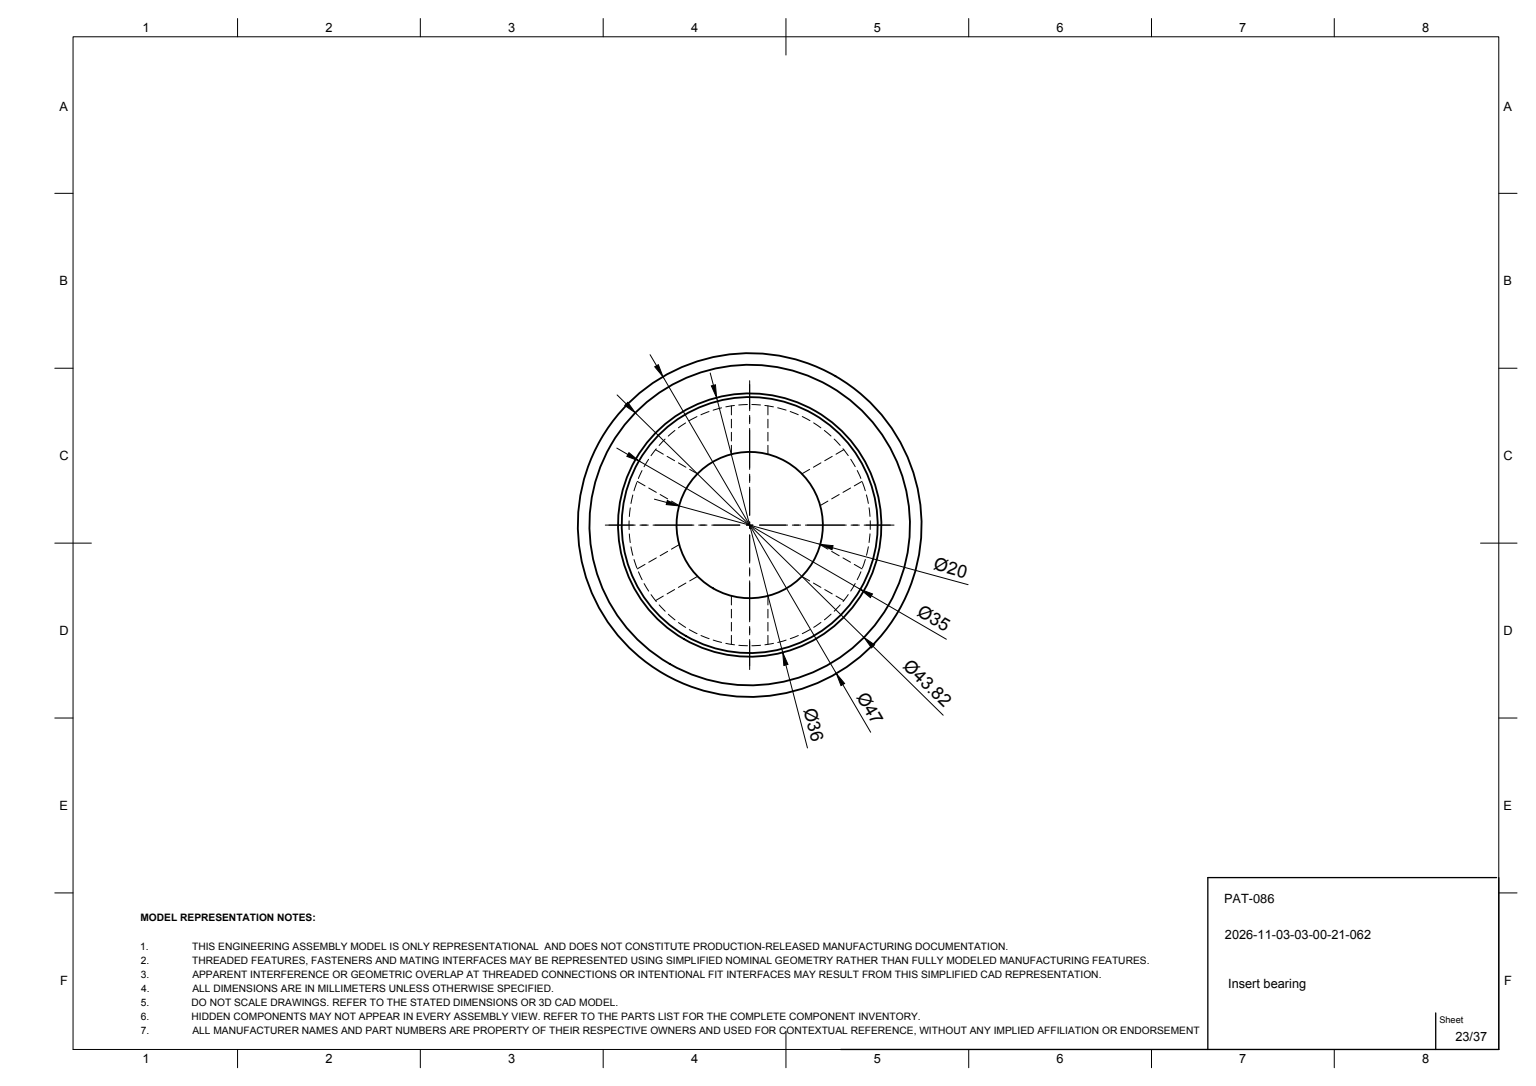
ISO-10303-21;
HEADER;
/* Generated by software containing ST-Developer
 * from STEP Tools, Inc. (www.steptools.com) 
 */

FILE_DESCRIPTION(
/* description */ ('Ratchet and pawl hand winch drum'),
/* implementation_level */ '2;1');

FILE_NAME(
/* name */ 'Insert bearing.step',
/* time_stamp */ '2026-10-27T12:42:58-07:00',
/* author */ (''),
/* organization */ (''),
/* preprocessor_version */ 'ST-DEVELOPER v20.2',
/* originating_system */ 'Autodesk Translation Framework v15.17.0.0',
/* authorisation */ '');

FILE_SCHEMA (('AUTOMOTIVE_DESIGN { 1 0 10303 214 3 1 1 }'));
ENDSEC;

DATA;
#10=MECHANICAL_DESIGN_GEOMETRIC_PRESENTATION_REPRESENTATION('',(#405,#406),#11801);
#273=B_SPLINE_CURVE_WITH_KNOTS('',3,(#9945,#9946,#9947,#9948,#9949,#9950,
#9951,#9952,#9953,#9954),.UNSPECIFIED.,.F.,.F.,(4,2,2,2,4),(1.13193471301885,
1.22626174930539,1.32058878559194,1.41491753480854,1.50924628402513),
 .UNSPECIFIED.);
#274=B_SPLINE_CURVE_WITH_KNOTS('',3,(#9956,#9957,#9958,#9959,#9960,#9961,
#9962,#9963,#9964,#9965,#9966,#9967,#9968,#9969,#9970,#9971,#9972,#9973),
 .UNSPECIFIED.,.F.,.F.,(4,2,2,2,2,2,2,2,4),(0.377311571006283,0.471638607292829,
0.565965643579376,0.66029439279597,0.754623142012565,0.84895189122916,0.943280640445754,
1.0376076767323,1.13193471301885),.UNSPECIFIED.);
#275=B_SPLINE_CURVE_WITH_KNOTS('',3,(#9974,#9975,#9976,#9977,#9978,#9979,
#9980,#9981,#9982,#9983),.UNSPECIFIED.,.F.,.F.,(4,2,2,2,4),(1.50924628402513,
1.60357503324173,1.69790378245832,1.79223081874487,1.88655785503141),
 .UNSPECIFIED.);
#276=B_SPLINE_CURVE_WITH_KNOTS('',3,(#9986,#9987,#9988,#9989,#9990,#9991,
#9992,#9993,#9994,#9995,#9996,#9997,#9998,#9999,#10000,#10001,#10002,#10003,
#10004,#10005,#10006,#10007,#10008,#10009,#10010,#10011,#10012,#10013,#10014,
#10015,#10016,#10017,#10018,#10019),.UNSPECIFIED.,.T.,.F.,(4,2,2,2,2,2,
2,2,2,2,2,2,2,2,2,2,4),(0.,0.0946120580087934,0.189224116017587,0.283822945575014,
0.378421775132442,0.47302060468987,0.567619434247297,0.662231492256091,
0.756843550264884,0.851455608273677,0.94606766628247,1.0406664958399,1.13526532539733,
1.22986415495475,1.32446298451218,1.41907504252097,1.51368710052977),
 .UNSPECIFIED.);
#277=B_SPLINE_CURVE_WITH_KNOTS('',3,(#10022,#10023,#10024,#10025,#10026,
#10027,#10028,#10029,#10030,#10031,#10032,#10033,#10034,#10035,#10036,#10037,
#10038,#10039,#10040,#10041,#10042,#10043,#10044,#10045,#10046,#10047,#10048,
#10049,#10050,#10051,#10052,#10053,#10054,#10055),.UNSPECIFIED.,.T.,.F.,
(4,2,2,2,2,2,2,2,2,2,2,2,2,2,2,2,4),(0.,0.0946120580087934,0.189224116017587,
0.283822945575014,0.378421775132442,0.47302060468987,0.567619434247297,
0.66223149225609,0.756843550264884,0.851455608273677,0.94606766628247,1.0406664958399,
1.13526532539733,1.22986415495475,1.32446298451218,1.41907504252097,1.51368710052977),
 .UNSPECIFIED.);
#278=B_SPLINE_CURVE_WITH_KNOTS('',3,(#10059,#10060,#10061,#10062,#10063,
#10064,#10065,#10066,#10067,#10068),.UNSPECIFIED.,.F.,.F.,(4,2,2,2,4),(1.13193471301885,
1.22626174930539,1.32058878559194,1.41491753480854,1.50924628402513),
 .UNSPECIFIED.);
#279=B_SPLINE_CURVE_WITH_KNOTS('',3,(#10070,#10071,#10072,#10073,#10074,
#10075,#10076,#10077,#10078,#10079,#10080,#10081,#10082,#10083,#10084,#10085,
#10086,#10087),.UNSPECIFIED.,.F.,.F.,(4,2,2,2,2,2,2,2,4),(0.377311571006283,
0.47163860729283,0.565965643579376,0.660294392795971,0.754623142012565,
0.84895189122916,0.943280640445755,1.0376076767323,1.13193471301885),
 .UNSPECIFIED.);
#280=B_SPLINE_CURVE_WITH_KNOTS('',3,(#10088,#10089,#10090,#10091,#10092,
#10093,#10094,#10095,#10096,#10097),.UNSPECIFIED.,.F.,.F.,(4,2,2,2,4),(1.50924628402513,
1.60357503324173,1.69790378245832,1.79223081874487,1.88655785503141),
 .UNSPECIFIED.);
#281=B_SPLINE_CURVE_WITH_KNOTS('',3,(#10106,#10107,#10108,#10109,#10110,
#10111,#10112,#10113,#10114,#10115,#10116,#10117,#10118,#10119,#10120,#10121,
#10122,#10123),.UNSPECIFIED.,.F.,.F.,(4,2,2,2,2,2,2,2,4),(0.377311571006282,
0.471638607292829,0.565965643579376,0.660294392795971,0.754623142012565,
0.84895189122916,0.943280640445754,1.0376076767323,1.13193471301885),
 .UNSPECIFIED.);
#282=B_SPLINE_CURVE_WITH_KNOTS('',3,(#10125,#10126,#10127,#10128,#10129,
#10130,#10131,#10132,#10133,#10134),.UNSPECIFIED.,.F.,.F.,(4,2,2,2,4),(1.13193471301885,
1.22626174930539,1.32058878559194,1.41491753480854,1.50924628402513),
 .UNSPECIFIED.);
#283=B_SPLINE_CURVE_WITH_KNOTS('',3,(#10135,#10136,#10137,#10138,#10139,
#10140,#10141,#10142,#10143,#10144),.UNSPECIFIED.,.F.,.F.,(4,2,2,2,4),(1.50924628402513,
1.60357503324172,1.69790378245832,1.79223081874487,1.88655785503141),
 .UNSPECIFIED.);
#284=B_SPLINE_CURVE_WITH_KNOTS('',3,(#10147,#10148,#10149,#10150,#10151,
#10152,#10153,#10154,#10155,#10156,#10157,#10158,#10159,#10160,#10161,#10162,
#10163,#10164),.UNSPECIFIED.,.F.,.F.,(4,2,2,2,2,2,2,2,4),(0.377311571006283,
0.47163860729283,0.565965643579376,0.660294392795971,0.754623142012565,
0.84895189122916,0.943280640445754,1.0376076767323,1.13193471301885),
 .UNSPECIFIED.);
#285=B_SPLINE_CURVE_WITH_KNOTS('',3,(#10166,#10167,#10168,#10169,#10170,
#10171,#10172,#10173,#10174,#10175),.UNSPECIFIED.,.F.,.F.,(4,2,2,2,4),(1.13193471301885,
1.22626174930539,1.32058878559194,1.41491753480854,1.50924628402513),
 .UNSPECIFIED.);
#286=B_SPLINE_CURVE_WITH_KNOTS('',3,(#10176,#10177,#10178,#10179,#10180,
#10181,#10182,#10183,#10184,#10185),.UNSPECIFIED.,.F.,.F.,(4,2,2,2,4),(1.50924628402513,
1.60357503324173,1.69790378245832,1.79223081874487,1.88655785503141),
 .UNSPECIFIED.);
#287=B_SPLINE_CURVE_WITH_KNOTS('',3,(#10188,#10189,#10190,#10191,#10192,
#10193,#10194,#10195,#10196,#10197,#10198,#10199,#10200,#10201,#10202,#10203,
#10204,#10205),.UNSPECIFIED.,.F.,.F.,(4,2,2,2,2,2,2,2,4),(0.377311571006282,
0.471638607292829,0.565965643579376,0.66029439279597,0.754623142012565,
0.84895189122916,0.943280640445754,1.0376076767323,1.13193471301885),
 .UNSPECIFIED.);
#288=B_SPLINE_CURVE_WITH_KNOTS('',3,(#10207,#10208,#10209,#10210,#10211,
#10212,#10213,#10214,#10215,#10216),.UNSPECIFIED.,.F.,.F.,(4,2,2,2,4),(1.13193471301885,
1.22626174930539,1.32058878559194,1.41491753480854,1.50924628402513),
 .UNSPECIFIED.);
#289=B_SPLINE_CURVE_WITH_KNOTS('',3,(#10217,#10218,#10219,#10220,#10221,
#10222,#10223,#10224,#10225,#10226),.UNSPECIFIED.,.F.,.F.,(4,2,2,2,4),(1.50924628402513,
1.60357503324172,1.69790378245832,1.79223081874487,1.88655785503141),
 .UNSPECIFIED.);
#290=B_SPLINE_CURVE_WITH_KNOTS('',3,(#10229,#10230,#10231,#10232,#10233,
#10234,#10235,#10236,#10237,#10238,#10239,#10240,#10241,#10242,#10243,#10244,
#10245,#10246),.UNSPECIFIED.,.F.,.F.,(4,2,2,2,2,2,2,2,4),(0.377311571006283,
0.471638607292829,0.565965643579376,0.660294392795971,0.754623142012565,
0.84895189122916,0.943280640445755,1.0376076767323,1.13193471301885),
 .UNSPECIFIED.);
#291=B_SPLINE_CURVE_WITH_KNOTS('',3,(#10248,#10249,#10250,#10251,#10252,
#10253,#10254,#10255,#10256,#10257),.UNSPECIFIED.,.F.,.F.,(4,2,2,2,4),(1.13193471301885,
1.22626174930539,1.32058878559194,1.41491753480854,1.50924628402513),
 .UNSPECIFIED.);
#292=B_SPLINE_CURVE_WITH_KNOTS('',3,(#10258,#10259,#10260,#10261,#10262,
#10263,#10264,#10265,#10266,#10267),.UNSPECIFIED.,.F.,.F.,(4,2,2,2,4),(1.50924628402513,
1.60357503324172,1.69790378245832,1.79223081874487,1.88655785503141),
 .UNSPECIFIED.);
#293=B_SPLINE_CURVE_WITH_KNOTS('',3,(#10271,#10272,#10273,#10274,#10275,
#10276,#10277,#10278,#10279,#10280,#10281,#10282,#10283,#10284,#10285,#10286,
#10287,#10288,#10289,#10290,#10291,#10292,#10293,#10294,#10295,#10296,#10297,
#10298,#10299,#10300,#10301,#10302,#10303,#10304),.UNSPECIFIED.,.T.,.F.,
(4,2,2,2,2,2,2,2,2,2,2,2,2,2,2,2,4),(0.,0.0946120580087934,0.189224116017587,
0.283822945575014,0.378421775132442,0.47302060468987,0.567619434247297,
0.66223149225609,0.756843550264884,0.851455608273677,0.94606766628247,1.0406664958399,
1.13526532539733,1.22986415495475,1.32446298451218,1.41907504252097,1.51368710052977),
 .UNSPECIFIED.);
#294=B_SPLINE_CURVE_WITH_KNOTS('',3,(#10307,#10308,#10309,#10310,#10311,
#10312,#10313,#10314,#10315,#10316,#10317,#10318,#10319,#10320,#10321,#10322,
#10323,#10324,#10325,#10326,#10327,#10328,#10329,#10330,#10331,#10332,#10333,
#10334,#10335,#10336,#10337,#10338,#10339,#10340),.UNSPECIFIED.,.T.,.F.,
(4,2,2,2,2,2,2,2,2,2,2,2,2,2,2,2,4),(0.,0.0946120580087934,0.189224116017587,
0.283822945575014,0.378421775132442,0.47302060468987,0.567619434247297,
0.66223149225609,0.756843550264884,0.851455608273677,0.94606766628247,1.0406664958399,
1.13526532539733,1.22986415495475,1.32446298451218,1.41907504252097,1.51368710052977),
 .UNSPECIFIED.);
#295=B_SPLINE_CURVE_WITH_KNOTS('',3,(#10345,#10346,#10347,#10348,#10349,
#10350,#10351,#10352,#10353,#10354,#10355,#10356,#10357,#10358,#10359,#10360,
#10361,#10362,#10363,#10364,#10365,#10366,#10367,#10368,#10369,#10370,#10371,
#10372,#10373,#10374,#10375,#10376,#10377,#10378),.UNSPECIFIED.,.T.,.F.,
(4,2,2,2,2,2,2,2,2,2,2,2,2,2,2,2,4),(0.,0.0946120580087934,0.189224116017587,
0.283822945575014,0.378421775132442,0.47302060468987,0.567619434247297,
0.66223149225609,0.756843550264884,0.851455608273677,0.94606766628247,1.0406664958399,
1.13526532539733,1.22986415495475,1.32446298451218,1.41907504252097,1.51368710052977),
 .UNSPECIFIED.);
#296=B_SPLINE_CURVE_WITH_KNOTS('',3,(#10381,#10382,#10383,#10384,#10385,
#10386,#10387,#10388,#10389,#10390,#10391,#10392,#10393,#10394,#10395,#10396,
#10397,#10398,#10399,#10400,#10401,#10402,#10403,#10404,#10405,#10406,#10407,
#10408,#10409,#10410,#10411,#10412,#10413,#10414),.UNSPECIFIED.,.T.,.F.,
(4,2,2,2,2,2,2,2,2,2,2,2,2,2,2,2,4),(0.,0.0946120580087934,0.189224116017587,
0.283822945575014,0.378421775132442,0.47302060468987,0.567619434247297,
0.66223149225609,0.756843550264884,0.851455608273677,0.94606766628247,1.0406664958399,
1.13526532539733,1.22986415495475,1.32446298451218,1.41907504252097,1.51368710052977),
 .UNSPECIFIED.);
#320=SPHERICAL_SURFACE('',#6968,2.35);
#337=SHAPE_REPRESENTATION_RELATIONSHIP('SRR','None',#11964,#371);
#371=ADVANCED_BREP_SHAPE_REPRESENTATION('',(#440,#441),#11781);
#405=STYLED_ITEM('',(#12213),#440);
#406=STYLED_ITEM('',(#12213),#441);
#440=MANIFOLD_SOLID_BREP('Body1',#6282);
#441=MANIFOLD_SOLID_BREP('Body2',#6283);
#541=FACE_BOUND('',#1434,.T.);
#542=FACE_BOUND('',#1436,.T.);
#543=FACE_BOUND('',#1437,.T.);
#544=FACE_BOUND('',#1439,.T.);
#545=FACE_BOUND('',#1443,.T.);
#546=FACE_BOUND('',#1444,.T.);
#547=FACE_BOUND('',#1445,.T.);
#548=FACE_BOUND('',#1446,.T.);
#549=FACE_BOUND('',#1447,.T.);
#550=FACE_BOUND('',#1448,.T.);
#551=FACE_BOUND('',#1454,.T.);
#552=FACE_BOUND('',#1456,.T.);
#553=FACE_BOUND('',#1459,.T.);
#554=FACE_BOUND('',#1461,.T.);
#555=FACE_BOUND('',#1462,.T.);
#556=FACE_BOUND('',#1463,.T.);
#557=FACE_BOUND('',#1464,.T.);
#558=FACE_BOUND('',#1465,.T.);
#559=FACE_BOUND('',#1466,.T.);
#697=PLANE('',#6966);
#698=PLANE('',#6971);
#699=PLANE('',#6981);
#700=PLANE('',#6983);
#701=PLANE('',#6987);
#991=FACE_OUTER_BOUND('',#1432,.T.);
#992=FACE_OUTER_BOUND('',#1433,.T.);
#993=FACE_OUTER_BOUND('',#1435,.T.);
#994=FACE_OUTER_BOUND('',#1438,.T.);
#995=FACE_OUTER_BOUND('',#1440,.T.);
#996=FACE_OUTER_BOUND('',#1441,.T.);
#997=FACE_OUTER_BOUND('',#1442,.T.);
#998=FACE_OUTER_BOUND('',#1449,.T.);
#999=FACE_OUTER_BOUND('',#1450,.T.);
#1000=FACE_OUTER_BOUND('',#1451,.T.);
#1001=FACE_OUTER_BOUND('',#1452,.T.);
#1002=FACE_OUTER_BOUND('',#1453,.T.);
#1003=FACE_OUTER_BOUND('',#1455,.T.);
#1004=FACE_OUTER_BOUND('',#1457,.T.);
#1005=FACE_OUTER_BOUND('',#1458,.T.);
#1006=FACE_OUTER_BOUND('',#1460,.T.);
#1432=EDGE_LOOP('',(#4879,#4880,#4881,#4882));
#1433=EDGE_LOOP('',(#4883));
#1434=EDGE_LOOP('',(#4884));
#1435=EDGE_LOOP('',(#4885,#4886));
#1436=EDGE_LOOP('',(#4887));
#1437=EDGE_LOOP('',(#4888));
#1438=EDGE_LOOP('',(#4889));
#1439=EDGE_LOOP('',(#4890));
#1440=EDGE_LOOP('',(#4891,#4892,#4893,#4894,#4895,#4896));
#1441=EDGE_LOOP('',(#4897,#4898,#4899,#4900,#4901,#4902));
#1442=EDGE_LOOP('',(#4903,#4904,#4905,#4906));
#1443=EDGE_LOOP('',(#4907,#4908,#4909));
#1444=EDGE_LOOP('',(#4910,#4911,#4912));
#1445=EDGE_LOOP('',(#4913,#4914,#4915));
#1446=EDGE_LOOP('',(#4916,#4917,#4918));
#1447=EDGE_LOOP('',(#4919,#4920,#4921));
#1448=EDGE_LOOP('',(#4922,#4923,#4924));
#1449=EDGE_LOOP('',(#4925,#4926,#4927,#4928,#4929,#4930));
#1450=EDGE_LOOP('',(#4931,#4932,#4933,#4934,#4935,#4936));
#1451=EDGE_LOOP('',(#4937,#4938,#4939,#4940,#4941,#4942));
#1452=EDGE_LOOP('',(#4943,#4944,#4945,#4946,#4947,#4948));
#1453=EDGE_LOOP('',(#4949));
#1454=EDGE_LOOP('',(#4950));
#1455=EDGE_LOOP('',(#4951));
#1456=EDGE_LOOP('',(#4952));
#1457=EDGE_LOOP('',(#4953,#4954,#4955,#4956));
#1458=EDGE_LOOP('',(#4957));
#1459=EDGE_LOOP('',(#4958));
#1460=EDGE_LOOP('',(#4959,#4960,#4961,#4962));
#1461=EDGE_LOOP('',(#4963));
#1462=EDGE_LOOP('',(#4964));
#1463=EDGE_LOOP('',(#4965));
#1464=EDGE_LOOP('',(#4966));
#1465=EDGE_LOOP('',(#4967));
#1466=EDGE_LOOP('',(#4968));
#1900=LINE('',#9930,#2411);
#1901=LINE('',#9985,#2412);
#1902=LINE('',#10057,#2413);
#1903=LINE('',#10102,#2414);
#1904=LINE('',#10270,#2415);
#1905=LINE('',#10341,#2416);
#1906=LINE('',#10344,#2417);
#1907=LINE('',#10415,#2418);
#1908=LINE('',#10425,#2419);
#1909=LINE('',#10430,#2420);
#2411=VECTOR('',#8133,1.8);
#2412=VECTOR('',#8150,0.25);
#2413=VECTOR('',#8153,0.25);
#2414=VECTOR('',#8158,1.65);
#2415=VECTOR('',#8163,0.25);
#2416=VECTOR('',#8166,0.25);
#2417=VECTOR('',#8169,0.25);
#2418=VECTOR('',#8172,0.25);
#2419=VECTOR('',#8185,1.75);
#2420=VECTOR('',#8192,1.);
#2832=CIRCLE('',#6964,1.8);
#2833=CIRCLE('',#6965,1.8);
#2834=CIRCLE('',#6967,2.19089023002066);
#2835=CIRCLE('',#6969,2.35);
#2836=CIRCLE('',#6970,2.19089023002066);
#2837=CIRCLE('',#6975,1.65);
#2838=CIRCLE('',#6976,1.65);
#2839=CIRCLE('',#6982,1.);
#2840=CIRCLE('',#6984,1.75);
#2841=CIRCLE('',#6986,1.75);
#2842=CIRCLE('',#6988,1.);
#3154=VERTEX_POINT('',#9927);
#3155=VERTEX_POINT('',#9929);
#3156=VERTEX_POINT('',#9933);
#3157=VERTEX_POINT('',#9936);
#3158=VERTEX_POINT('',#9937);
#3159=VERTEX_POINT('',#9939);
#3160=VERTEX_POINT('',#9943);
#3161=VERTEX_POINT('',#9944);
#3162=VERTEX_POINT('',#9955);
#3163=VERTEX_POINT('',#9984);
#3164=VERTEX_POINT('',#10021);
#3165=VERTEX_POINT('',#10056);
#3166=VERTEX_POINT('',#10058);
#3167=VERTEX_POINT('',#10069);
#3168=VERTEX_POINT('',#10099);
#3169=VERTEX_POINT('',#10101);
#3170=VERTEX_POINT('',#10104);
#3171=VERTEX_POINT('',#10105);
#3172=VERTEX_POINT('',#10124);
#3173=VERTEX_POINT('',#10145);
#3174=VERTEX_POINT('',#10146);
#3175=VERTEX_POINT('',#10165);
#3176=VERTEX_POINT('',#10186);
#3177=VERTEX_POINT('',#10187);
#3178=VERTEX_POINT('',#10206);
#3179=VERTEX_POINT('',#10227);
#3180=VERTEX_POINT('',#10228);
#3181=VERTEX_POINT('',#10247);
#3182=VERTEX_POINT('',#10269);
#3183=VERTEX_POINT('',#10306);
#3184=VERTEX_POINT('',#10343);
#3185=VERTEX_POINT('',#10380);
#3186=VERTEX_POINT('',#10417);
#3187=VERTEX_POINT('',#10420);
#3188=VERTEX_POINT('',#10423);
#3189=VERTEX_POINT('',#10427);
#3783=EDGE_CURVE('',#3154,#3154,#2832,.T.);
#3784=EDGE_CURVE('',#3154,#3155,#1900,.T.);
#3785=EDGE_CURVE('',#3155,#3155,#2833,.T.);
#3786=EDGE_CURVE('',#3156,#3156,#2834,.T.);
#3787=EDGE_CURVE('',#3157,#3158,#2835,.T.);
#3788=EDGE_CURVE('',#3159,#3159,#2836,.T.);
#3789=EDGE_CURVE('',#3160,#3161,#273,.T.);
#3790=EDGE_CURVE('',#3162,#3160,#274,.T.);
#3791=EDGE_CURVE('',#3161,#3162,#275,.T.);
#3792=EDGE_CURVE('',#3161,#3163,#1901,.T.);
#3793=EDGE_CURVE('',#3163,#3163,#276,.T.);
#3794=EDGE_CURVE('',#3164,#3164,#277,.T.);
#3795=EDGE_CURVE('',#3164,#3165,#1902,.T.);
#3796=EDGE_CURVE('',#3166,#3165,#278,.T.);
#3797=EDGE_CURVE('',#3167,#3166,#279,.T.);
#3798=EDGE_CURVE('',#3165,#3167,#280,.T.);
#3799=EDGE_CURVE('',#3168,#3168,#2837,.T.);
#3800=EDGE_CURVE('',#3168,#3169,#1903,.T.);
#3801=EDGE_CURVE('',#3169,#3169,#2838,.T.);
#3802=EDGE_CURVE('',#3170,#3171,#281,.T.);
#3803=EDGE_CURVE('',#3171,#3172,#282,.T.);
#3804=EDGE_CURVE('',#3172,#3170,#283,.T.);
#3805=EDGE_CURVE('',#3173,#3174,#284,.T.);
#3806=EDGE_CURVE('',#3174,#3175,#285,.T.);
#3807=EDGE_CURVE('',#3175,#3173,#286,.T.);
#3808=EDGE_CURVE('',#3176,#3177,#287,.T.);
#3809=EDGE_CURVE('',#3177,#3178,#288,.T.);
#3810=EDGE_CURVE('',#3178,#3176,#289,.T.);
#3811=EDGE_CURVE('',#3179,#3180,#290,.T.);
#3812=EDGE_CURVE('',#3180,#3181,#291,.T.);
#3813=EDGE_CURVE('',#3181,#3179,#292,.T.);
#3814=EDGE_CURVE('',#3172,#3182,#1904,.T.);
#3815=EDGE_CURVE('',#3182,#3182,#293,.T.);
#3816=EDGE_CURVE('',#3183,#3183,#294,.T.);
#3817=EDGE_CURVE('',#3183,#3175,#1905,.T.);
#3818=EDGE_CURVE('',#3178,#3184,#1906,.T.);
#3819=EDGE_CURVE('',#3184,#3184,#295,.T.);
#3820=EDGE_CURVE('',#3185,#3185,#296,.T.);
#3821=EDGE_CURVE('',#3185,#3181,#1907,.T.);
#3822=EDGE_CURVE('',#3186,#3186,#2839,.T.);
#3823=EDGE_CURVE('',#3187,#3187,#2840,.T.);
#3824=EDGE_CURVE('',#3188,#3188,#2841,.T.);
#3825=EDGE_CURVE('',#3188,#3187,#1908,.T.);
#3826=EDGE_CURVE('',#3189,#3189,#2842,.T.);
#3827=EDGE_CURVE('',#3189,#3186,#1909,.T.);
#4879=ORIENTED_EDGE('',*,*,#3783,.T.);
#4880=ORIENTED_EDGE('',*,*,#3784,.T.);
#4881=ORIENTED_EDGE('',*,*,#3785,.F.);
#4882=ORIENTED_EDGE('',*,*,#3784,.F.);
#4883=ORIENTED_EDGE('',*,*,#3786,.F.);
#4884=ORIENTED_EDGE('',*,*,#3785,.T.);
#4885=ORIENTED_EDGE('',*,*,#3787,.T.);
#4886=ORIENTED_EDGE('',*,*,#3787,.F.);
#4887=ORIENTED_EDGE('',*,*,#3786,.T.);
#4888=ORIENTED_EDGE('',*,*,#3788,.F.);
#4889=ORIENTED_EDGE('',*,*,#3788,.T.);
#4890=ORIENTED_EDGE('',*,*,#3783,.F.);
#4891=ORIENTED_EDGE('',*,*,#3789,.F.);
#4892=ORIENTED_EDGE('',*,*,#3790,.F.);
#4893=ORIENTED_EDGE('',*,*,#3791,.F.);
#4894=ORIENTED_EDGE('',*,*,#3792,.T.);
#4895=ORIENTED_EDGE('',*,*,#3793,.F.);
#4896=ORIENTED_EDGE('',*,*,#3792,.F.);
#4897=ORIENTED_EDGE('',*,*,#3794,.F.);
#4898=ORIENTED_EDGE('',*,*,#3795,.T.);
#4899=ORIENTED_EDGE('',*,*,#3796,.F.);
#4900=ORIENTED_EDGE('',*,*,#3797,.F.);
#4901=ORIENTED_EDGE('',*,*,#3798,.F.);
#4902=ORIENTED_EDGE('',*,*,#3795,.F.);
#4903=ORIENTED_EDGE('',*,*,#3799,.F.);
#4904=ORIENTED_EDGE('',*,*,#3800,.T.);
#4905=ORIENTED_EDGE('',*,*,#3801,.T.);
#4906=ORIENTED_EDGE('',*,*,#3800,.F.);
#4907=ORIENTED_EDGE('',*,*,#3790,.T.);
#4908=ORIENTED_EDGE('',*,*,#3789,.T.);
#4909=ORIENTED_EDGE('',*,*,#3791,.T.);
#4910=ORIENTED_EDGE('',*,*,#3797,.T.);
#4911=ORIENTED_EDGE('',*,*,#3796,.T.);
#4912=ORIENTED_EDGE('',*,*,#3798,.T.);
#4913=ORIENTED_EDGE('',*,*,#3802,.T.);
#4914=ORIENTED_EDGE('',*,*,#3803,.T.);
#4915=ORIENTED_EDGE('',*,*,#3804,.T.);
#4916=ORIENTED_EDGE('',*,*,#3805,.T.);
#4917=ORIENTED_EDGE('',*,*,#3806,.T.);
#4918=ORIENTED_EDGE('',*,*,#3807,.T.);
#4919=ORIENTED_EDGE('',*,*,#3808,.T.);
#4920=ORIENTED_EDGE('',*,*,#3809,.T.);
#4921=ORIENTED_EDGE('',*,*,#3810,.T.);
#4922=ORIENTED_EDGE('',*,*,#3811,.T.);
#4923=ORIENTED_EDGE('',*,*,#3812,.T.);
#4924=ORIENTED_EDGE('',*,*,#3813,.T.);
#4925=ORIENTED_EDGE('',*,*,#3803,.F.);
#4926=ORIENTED_EDGE('',*,*,#3802,.F.);
#4927=ORIENTED_EDGE('',*,*,#3804,.F.);
#4928=ORIENTED_EDGE('',*,*,#3814,.T.);
#4929=ORIENTED_EDGE('',*,*,#3815,.F.);
#4930=ORIENTED_EDGE('',*,*,#3814,.F.);
#4931=ORIENTED_EDGE('',*,*,#3816,.F.);
#4932=ORIENTED_EDGE('',*,*,#3817,.T.);
#4933=ORIENTED_EDGE('',*,*,#3806,.F.);
#4934=ORIENTED_EDGE('',*,*,#3805,.F.);
#4935=ORIENTED_EDGE('',*,*,#3807,.F.);
#4936=ORIENTED_EDGE('',*,*,#3817,.F.);
#4937=ORIENTED_EDGE('',*,*,#3809,.F.);
#4938=ORIENTED_EDGE('',*,*,#3808,.F.);
#4939=ORIENTED_EDGE('',*,*,#3810,.F.);
#4940=ORIENTED_EDGE('',*,*,#3818,.T.);
#4941=ORIENTED_EDGE('',*,*,#3819,.F.);
#4942=ORIENTED_EDGE('',*,*,#3818,.F.);
#4943=ORIENTED_EDGE('',*,*,#3820,.F.);
#4944=ORIENTED_EDGE('',*,*,#3821,.T.);
#4945=ORIENTED_EDGE('',*,*,#3812,.F.);
#4946=ORIENTED_EDGE('',*,*,#3811,.F.);
#4947=ORIENTED_EDGE('',*,*,#3813,.F.);
#4948=ORIENTED_EDGE('',*,*,#3821,.F.);
#4949=ORIENTED_EDGE('',*,*,#3801,.F.);
#4950=ORIENTED_EDGE('',*,*,#3822,.T.);
#4951=ORIENTED_EDGE('',*,*,#3823,.F.);
#4952=ORIENTED_EDGE('',*,*,#3799,.T.);
#4953=ORIENTED_EDGE('',*,*,#3824,.F.);
#4954=ORIENTED_EDGE('',*,*,#3825,.T.);
#4955=ORIENTED_EDGE('',*,*,#3823,.T.);
#4956=ORIENTED_EDGE('',*,*,#3825,.F.);
#4957=ORIENTED_EDGE('',*,*,#3824,.T.);
#4958=ORIENTED_EDGE('',*,*,#3826,.F.);
#4959=ORIENTED_EDGE('',*,*,#3826,.T.);
#4960=ORIENTED_EDGE('',*,*,#3827,.T.);
#4961=ORIENTED_EDGE('',*,*,#3822,.F.);
#4962=ORIENTED_EDGE('',*,*,#3827,.F.);
#4963=ORIENTED_EDGE('',*,*,#3794,.T.);
#4964=ORIENTED_EDGE('',*,*,#3793,.T.);
#4965=ORIENTED_EDGE('',*,*,#3816,.T.);
#4966=ORIENTED_EDGE('',*,*,#3815,.T.);
#4967=ORIENTED_EDGE('',*,*,#3820,.T.);
#4968=ORIENTED_EDGE('',*,*,#3819,.T.);
#5861=CYLINDRICAL_SURFACE('',#6963,1.8);
#5862=CYLINDRICAL_SURFACE('',#6972,0.25);
#5863=CYLINDRICAL_SURFACE('',#6973,0.25);
#5864=CYLINDRICAL_SURFACE('',#6974,1.65);
#5865=CYLINDRICAL_SURFACE('',#6977,0.25);
#5866=CYLINDRICAL_SURFACE('',#6978,0.25);
#5867=CYLINDRICAL_SURFACE('',#6979,0.25);
#5868=CYLINDRICAL_SURFACE('',#6980,0.25);
#5869=CYLINDRICAL_SURFACE('',#6985,1.75);
#5870=CYLINDRICAL_SURFACE('',#6989,1.);
#6061=ADVANCED_FACE('',(#991),#5861,.F.);
#6062=ADVANCED_FACE('',(#992,#541),#697,.T.);
#6063=ADVANCED_FACE('',(#993,#542,#543),#320,.T.);
#6064=ADVANCED_FACE('',(#994,#544),#698,.T.);
#6065=ADVANCED_FACE('',(#995),#5862,.F.);
#6066=ADVANCED_FACE('',(#996),#5863,.F.);
#6067=ADVANCED_FACE('',(#997,#545,#546,#547,#548,#549,#550),#5864,.T.);
#6068=ADVANCED_FACE('',(#998),#5865,.F.);
#6069=ADVANCED_FACE('',(#999),#5866,.F.);
#6070=ADVANCED_FACE('',(#1000),#5867,.F.);
#6071=ADVANCED_FACE('',(#1001),#5868,.F.);
#6072=ADVANCED_FACE('',(#1002,#551),#699,.T.);
#6073=ADVANCED_FACE('',(#1003,#552),#700,.T.);
#6074=ADVANCED_FACE('',(#1004),#5869,.T.);
#6075=ADVANCED_FACE('',(#1005,#553),#701,.T.);
#6076=ADVANCED_FACE('',(#1006,#554,#555,#556,#557,#558,#559),#5870,.F.);
#6282=CLOSED_SHELL('',(#6061,#6062,#6063,#6064));
#6283=CLOSED_SHELL('',(#6065,#6066,#6067,#6068,#6069,#6070,#6071,#6072,
#6073,#6074,#6075,#6076));
#6962=AXIS2_PLACEMENT_3D('',#9925,#8127,#8128);
#6963=AXIS2_PLACEMENT_3D('',#9926,#8129,#8130);
#6964=AXIS2_PLACEMENT_3D('',#9928,#8131,#8132);
#6965=AXIS2_PLACEMENT_3D('',#9931,#8134,#8135);
#6966=AXIS2_PLACEMENT_3D('',#9932,#8136,#8137);
#6967=AXIS2_PLACEMENT_3D('',#9934,#8138,#8139);
#6968=AXIS2_PLACEMENT_3D('',#9935,#8140,#8141);
#6969=AXIS2_PLACEMENT_3D('',#9938,#8142,#8143);
#6970=AXIS2_PLACEMENT_3D('',#9940,#8144,#8145);
#6971=AXIS2_PLACEMENT_3D('',#9941,#8146,#8147);
#6972=AXIS2_PLACEMENT_3D('',#9942,#8148,#8149);
#6973=AXIS2_PLACEMENT_3D('',#10020,#8151,#8152);
#6974=AXIS2_PLACEMENT_3D('',#10098,#8154,#8155);
#6975=AXIS2_PLACEMENT_3D('',#10100,#8156,#8157);
#6976=AXIS2_PLACEMENT_3D('',#10103,#8159,#8160);
#6977=AXIS2_PLACEMENT_3D('',#10268,#8161,#8162);
#6978=AXIS2_PLACEMENT_3D('',#10305,#8164,#8165);
#6979=AXIS2_PLACEMENT_3D('',#10342,#8167,#8168);
#6980=AXIS2_PLACEMENT_3D('',#10379,#8170,#8171);
#6981=AXIS2_PLACEMENT_3D('',#10416,#8173,#8174);
#6982=AXIS2_PLACEMENT_3D('',#10418,#8175,#8176);
#6983=AXIS2_PLACEMENT_3D('',#10419,#8177,#8178);
#6984=AXIS2_PLACEMENT_3D('',#10421,#8179,#8180);
#6985=AXIS2_PLACEMENT_3D('',#10422,#8181,#8182);
#6986=AXIS2_PLACEMENT_3D('',#10424,#8183,#8184);
#6987=AXIS2_PLACEMENT_3D('',#10426,#8186,#8187);
#6988=AXIS2_PLACEMENT_3D('',#10428,#8188,#8189);
#6989=AXIS2_PLACEMENT_3D('',#10429,#8190,#8191);
#8127=DIRECTION('axis',(0.,0.,1.));
#8128=DIRECTION('refdir',(1.,0.,0.));
#8129=DIRECTION('center_axis',(0.,-1.,0.));
#8130=DIRECTION('ref_axis',(1.,0.,0.));
#8131=DIRECTION('center_axis',(0.,-1.,0.));
#8132=DIRECTION('ref_axis',(1.,0.,0.));
#8133=DIRECTION('',(0.,1.,0.));
#8134=DIRECTION('center_axis',(0.,-1.,0.));
#8135=DIRECTION('ref_axis',(1.,0.,0.));
#8136=DIRECTION('center_axis',(0.,1.,0.));
#8137=DIRECTION('ref_axis',(0.,0.,1.));
#8138=DIRECTION('center_axis',(0.,-1.,0.));
#8139=DIRECTION('ref_axis',(1.,0.,0.));
#8140=DIRECTION('center_axis',(6.12323399573677E-17,0.,1.));
#8141=DIRECTION('ref_axis',(1.,0.,0.));
#8142=DIRECTION('center_axis',(1.22464679914735E-16,-1.,0.));
#8143=DIRECTION('ref_axis',(-1.,-1.22464679914735E-16,0.));
#8144=DIRECTION('center_axis',(0.,-1.,0.));
#8145=DIRECTION('ref_axis',(1.,0.,0.));
#8146=DIRECTION('center_axis',(0.,-1.,0.));
#8147=DIRECTION('ref_axis',(0.,0.,-1.));
#8148=DIRECTION('center_axis',(-0.866025403784438,0.,-0.5));
#8149=DIRECTION('ref_axis',(-0.5,0.,0.866025403784438));
#8150=DIRECTION('',(-0.866025403784438,0.,-0.5));
#8151=DIRECTION('center_axis',(-0.866025403784438,0.,-0.5));
#8152=DIRECTION('ref_axis',(-0.5,0.,0.866025403784438));
#8153=DIRECTION('',(-0.866025403784438,0.,-0.5));
#8154=DIRECTION('center_axis',(0.,-1.,0.));
#8155=DIRECTION('ref_axis',(1.,0.,0.));
#8156=DIRECTION('center_axis',(0.,-1.,0.));
#8157=DIRECTION('ref_axis',(1.,0.,0.));
#8158=DIRECTION('',(0.,1.,0.));
#8159=DIRECTION('center_axis',(0.,-1.,0.));
#8160=DIRECTION('ref_axis',(1.,0.,0.));
#8161=DIRECTION('center_axis',(0.866025403784439,0.,-0.5));
#8162=DIRECTION('ref_axis',(-0.5,0.,-0.866025403784439));
#8163=DIRECTION('',(0.866025403784439,0.,-0.5));
#8164=DIRECTION('center_axis',(0.866025403784439,0.,-0.5));
#8165=DIRECTION('ref_axis',(-0.5,0.,-0.866025403784439));
#8166=DIRECTION('',(0.866025403784439,0.,-0.5));
#8167=DIRECTION('center_axis',(0.,0.,1.));
#8168=DIRECTION('ref_axis',(1.,0.,0.));
#8169=DIRECTION('',(0.,0.,1.));
#8170=DIRECTION('center_axis',(0.,0.,1.));
#8171=DIRECTION('ref_axis',(1.,0.,0.));
#8172=DIRECTION('',(0.,0.,1.));
#8173=DIRECTION('center_axis',(0.,1.,0.));
#8174=DIRECTION('ref_axis',(0.,0.,1.));
#8175=DIRECTION('center_axis',(0.,-1.,0.));
#8176=DIRECTION('ref_axis',(1.,0.,0.));
#8177=DIRECTION('center_axis',(0.,1.,0.));
#8178=DIRECTION('ref_axis',(0.,0.,1.));
#8179=DIRECTION('center_axis',(0.,-1.,0.));
#8180=DIRECTION('ref_axis',(1.,0.,0.));
#8181=DIRECTION('center_axis',(0.,-1.,0.));
#8182=DIRECTION('ref_axis',(1.,0.,0.));
#8183=DIRECTION('center_axis',(0.,-1.,0.));
#8184=DIRECTION('ref_axis',(1.,0.,0.));
#8185=DIRECTION('',(0.,1.,0.));
#8186=DIRECTION('center_axis',(0.,-1.,0.));
#8187=DIRECTION('ref_axis',(0.,0.,-1.));
#8188=DIRECTION('center_axis',(0.,-1.,0.));
#8189=DIRECTION('ref_axis',(1.,0.,0.));
#8190=DIRECTION('center_axis',(0.,-1.,0.));
#8191=DIRECTION('ref_axis',(1.,0.,0.));
#8192=DIRECTION('',(0.,1.,0.));
#9925=CARTESIAN_POINT('',(0.,0.,0.));
#9926=CARTESIAN_POINT('Origin',(0.,0.,0.));
#9927=CARTESIAN_POINT('',(-1.8,-0.85,-2.20436423846524E-16));
#9928=CARTESIAN_POINT('Origin',(0.,-0.85,0.));
#9929=CARTESIAN_POINT('',(-1.8,0.85,-2.20436423846524E-16));
#9930=CARTESIAN_POINT('',(-1.8,0.,-2.20436423846524E-16));
#9931=CARTESIAN_POINT('Origin',(0.,0.85,0.));
#9932=CARTESIAN_POINT('Origin',(2.19089023002066,0.85,0.));
#9933=CARTESIAN_POINT('',(2.19089023002066,0.85,0.));
#9934=CARTESIAN_POINT('Origin',(0.,0.85,0.));
#9935=CARTESIAN_POINT('Origin',(3.99680288865056E-15,0.,0.));
#9936=CARTESIAN_POINT('',(3.85290688975075E-15,-1.76221774462768E-32,2.35));
#9937=CARTESIAN_POINT('',(3.85290688975075E-15,-1.76221774462768E-32,-2.35));
#9938=CARTESIAN_POINT('Origin',(3.99680288865056E-15,0.,0.));
#9939=CARTESIAN_POINT('',(2.19089023002066,-0.85,0.));
#9940=CARTESIAN_POINT('Origin',(0.,-0.85,0.));
#9941=CARTESIAN_POINT('Origin',(1.8,-0.85,0.));
#9942=CARTESIAN_POINT('Origin',(0.,1.55,0.));
#9943=CARTESIAN_POINT('',(1.42894191624432,1.8,0.825000000000001));
#9944=CARTESIAN_POINT('',(1.53744468918255,1.55,0.598968970568896));
#9945=CARTESIAN_POINT('Ctrl Pts',(1.42894191624432,1.8,0.825000000000001));
#9946=CARTESIAN_POINT('Ctrl Pts',(1.44466308895875,1.8,0.797770130104052));
#9947=CARTESIAN_POINT('Ctrl Pts',(1.46055812562105,1.79370633789704,0.768258557763732));
#9948=CARTESIAN_POINT('Ctrl Pts',(1.48824888379079,1.76817777258318,0.713138492740816));
#9949=CARTESIAN_POINT('Ctrl Pts',(1.50008999307766,1.74894552961493,0.687551581002689));
#9950=CARTESIAN_POINT('Ctrl Pts',(1.51812136280714,1.70460745840382,0.646764802471699));
#9951=CARTESIAN_POINT('Ctrl Pts',(1.52552758004446,1.67652816181843,0.628833667319578));
#9952=CARTESIAN_POINT('Ctrl Pts',(1.53516661651472,1.61494799959182,0.604921184808251));
#9953=CARTESIAN_POINT('Ctrl Pts',(1.53744468918255,1.58144291640553,0.598968970568896));
#9954=CARTESIAN_POINT('Ctrl Pts',(1.53744468918255,1.55,0.598968970568896));
#9955=CARTESIAN_POINT('',(1.42894191624432,1.3,0.825000000000001));
#9956=CARTESIAN_POINT('Ctrl Pts',(1.42894191624432,1.3,0.825000000000001));
#9957=CARTESIAN_POINT('Ctrl Pts',(1.4132207435299,1.3,0.852229869895949));
#9958=CARTESIAN_POINT('Ctrl Pts',(1.39561049050871,1.30629366210296,0.880751161609749));
#9959=CARTESIAN_POINT('Ctrl Pts',(1.36172049302549,1.33182222741682,0.932292094146256));
#9960=CARTESIAN_POINT('Ctrl Pts',(1.34548213209931,1.35105447038507,0.955340251466734));
#9961=CARTESIAN_POINT('Ctrl Pts',(1.31917543061769,1.39539254159618,0.99134926498299));
#9962=CARTESIAN_POINT('Ctrl Pts',(1.30734972067592,1.42347183818157,1.00672880483252));
#9963=CARTESIAN_POINT('Ctrl Pts',(1.29146042158868,1.48505200040818,1.02703269653942));
#9964=CARTESIAN_POINT('Ctrl Pts',(1.28744468918255,1.51855708359447,1.03198167246111));
#9965=CARTESIAN_POINT('Ctrl Pts',(1.28744468918255,1.58144291640553,1.03198167246111));
#9966=CARTESIAN_POINT('Ctrl Pts',(1.29146042158868,1.61494799959182,1.02703269653942));
#9967=CARTESIAN_POINT('Ctrl Pts',(1.30734972067592,1.67652816181843,1.00672880483252));
#9968=CARTESIAN_POINT('Ctrl Pts',(1.31917543061769,1.70460745840382,0.991349264982991));
#9969=CARTESIAN_POINT('Ctrl Pts',(1.34548213209931,1.74894552961493,0.955340251466735));
#9970=CARTESIAN_POINT('Ctrl Pts',(1.36172049302549,1.76817777258318,0.932292094146256));
#9971=CARTESIAN_POINT('Ctrl Pts',(1.39561049050871,1.79370633789704,0.880751161609749));
#9972=CARTESIAN_POINT('Ctrl Pts',(1.4132207435299,1.8,0.85222986989595));
#9973=CARTESIAN_POINT('Ctrl Pts',(1.42894191624432,1.8,0.825000000000001));
#9974=CARTESIAN_POINT('Ctrl Pts',(1.53744468918255,1.55,0.598968970568896));
#9975=CARTESIAN_POINT('Ctrl Pts',(1.53744468918255,1.51855708359447,0.598968970568896));
#9976=CARTESIAN_POINT('Ctrl Pts',(1.53516661651472,1.48505200040818,0.60492118480825));
#9977=CARTESIAN_POINT('Ctrl Pts',(1.52552758004446,1.42347183818157,0.628833667319578));
#9978=CARTESIAN_POINT('Ctrl Pts',(1.51812136280714,1.39539254159618,0.646764802471699));
#9979=CARTESIAN_POINT('Ctrl Pts',(1.50008999307766,1.35105447038507,0.687551581002689));
#9980=CARTESIAN_POINT('Ctrl Pts',(1.48824888379079,1.33182222741682,0.713138492740816));
#9981=CARTESIAN_POINT('Ctrl Pts',(1.46055812562105,1.30629366210296,0.768258557763732));
#9982=CARTESIAN_POINT('Ctrl Pts',(1.44466308895875,1.3,0.797770130104052));
#9983=CARTESIAN_POINT('Ctrl Pts',(1.42894191624432,1.3,0.825000000000001));
#9984=CARTESIAN_POINT('',(0.963525491562421,1.55,0.267616567329818));
#9985=CARTESIAN_POINT('',(0.125,1.55,-0.21650635094611));
#9986=CARTESIAN_POINT('Ctrl Pts',(0.963525491562421,1.55,0.267616567329818));
#9987=CARTESIAN_POINT('Ctrl Pts',(0.963525491562421,1.5815373526696,0.267616567329818));
#9988=CARTESIAN_POINT('Ctrl Pts',(0.961833761492987,1.61508042700263,0.273949373987484));
#9989=CARTESIAN_POINT('Ctrl Pts',(0.954308486908894,1.67663267125761,0.299111603474268));
#9990=CARTESIAN_POINT('Ctrl Pts',(0.948394987258249,1.70465411363682,0.31788699900678));
#9991=CARTESIAN_POINT('Ctrl Pts',(0.933155485613026,1.74889618382539,0.360174810895352));
#9992=CARTESIAN_POINT('Ctrl Pts',(0.92278792026947,1.76811531482682,0.386546956384144));
#9993=CARTESIAN_POINT('Ctrl Pts',(0.897143218189782,1.79367084275751,0.442820664919227));
#9994=CARTESIAN_POINT('Ctrl Pts',(0.881791875377343,1.8,0.472691670144998));
#9995=CARTESIAN_POINT('Ctrl Pts',(0.850258932191534,1.8,0.527308329855003));
#9996=CARTESIAN_POINT('Ctrl Pts',(0.832065554235658,1.79367084275751,0.555538485325664));
#9997=CARTESIAN_POINT('Ctrl Pts',(0.796153444118959,1.76811531482682,0.605884303066698));
#9998=CARTESIAN_POINT('Ctrl Pts',(0.778498278845144,1.74889618382539,0.62804895077401));
#9999=CARTESIAN_POINT('Ctrl Pts',(0.749495710301794,1.70465411363682,0.662390652284073));
#10000=CARTESIAN_POINT('Ctrl Pts',(0.73619249062986,1.67663267125761,0.676899590973058));
#10001=CARTESIAN_POINT('Ctrl Pts',(0.718163997970498,1.61508042700263,0.695997784676728));
#10002=CARTESIAN_POINT('Ctrl Pts',(0.713525491562421,1.5815373526696,0.700629269222037));
#10003=CARTESIAN_POINT('Ctrl Pts',(0.713525491562421,1.5184626473304,0.700629269222037));
#10004=CARTESIAN_POINT('Ctrl Pts',(0.718163997970498,1.48491957299737,0.695997784676728));
#10005=CARTESIAN_POINT('Ctrl Pts',(0.73619249062986,1.42336732874239,0.676899590973058));
#10006=CARTESIAN_POINT('Ctrl Pts',(0.749495710301794,1.39534588636318,0.662390652284073));
#10007=CARTESIAN_POINT('Ctrl Pts',(0.778498278845144,1.35110381617461,0.62804895077401));
#10008=CARTESIAN_POINT('Ctrl Pts',(0.796153444118959,1.33188468517318,0.605884303066698));
#10009=CARTESIAN_POINT('Ctrl Pts',(0.832065554235658,1.30632915724249,0.555538485325664));
#10010=CARTESIAN_POINT('Ctrl Pts',(0.850258932191534,1.3,0.527308329855003));
#10011=CARTESIAN_POINT('Ctrl Pts',(0.881791875377343,1.3,0.472691670144998));
#10012=CARTESIAN_POINT('Ctrl Pts',(0.897143218189782,1.30632915724249,0.442820664919227));
#10013=CARTESIAN_POINT('Ctrl Pts',(0.92278792026947,1.33188468517318,0.386546956384144));
#10014=CARTESIAN_POINT('Ctrl Pts',(0.933155485613026,1.35110381617461,0.360174810895352));
#10015=CARTESIAN_POINT('Ctrl Pts',(0.948394987258249,1.39534588636318,0.31788699900678));
#10016=CARTESIAN_POINT('Ctrl Pts',(0.954308486908894,1.42336732874239,0.299111603474268));
#10017=CARTESIAN_POINT('Ctrl Pts',(0.961833761492987,1.48491957299738,0.273949373987484));
#10018=CARTESIAN_POINT('Ctrl Pts',(0.963525491562421,1.5184626473304,0.267616567329818));
#10019=CARTESIAN_POINT('Ctrl Pts',(0.963525491562421,1.55,0.267616567329818));
#10020=CARTESIAN_POINT('Origin',(0.,1.55,0.));
#10021=CARTESIAN_POINT('',(-0.713525491562421,1.55,-0.700629269222037));
#10022=CARTESIAN_POINT('Ctrl Pts',(-0.713525491562421,1.55,-0.700629269222037));
#10023=CARTESIAN_POINT('Ctrl Pts',(-0.713525491562421,1.5184626473304,-0.700629269222037));
#10024=CARTESIAN_POINT('Ctrl Pts',(-0.718163997970498,1.48491957299737,
-0.695997784676728));
#10025=CARTESIAN_POINT('Ctrl Pts',(-0.73619249062986,1.42336732874239,-0.676899590973058));
#10026=CARTESIAN_POINT('Ctrl Pts',(-0.749495710301794,1.39534588636318,
-0.662390652284073));
#10027=CARTESIAN_POINT('Ctrl Pts',(-0.778498278845144,1.35110381617461,
-0.62804895077401));
#10028=CARTESIAN_POINT('Ctrl Pts',(-0.796153444118959,1.33188468517318,
-0.605884303066698));
#10029=CARTESIAN_POINT('Ctrl Pts',(-0.832065554235658,1.30632915724249,
-0.555538485325664));
#10030=CARTESIAN_POINT('Ctrl Pts',(-0.850258932191534,1.3,-0.527308329855003));
#10031=CARTESIAN_POINT('Ctrl Pts',(-0.881791875377343,1.3,-0.472691670144998));
#10032=CARTESIAN_POINT('Ctrl Pts',(-0.897143218189782,1.30632915724249,
-0.442820664919227));
#10033=CARTESIAN_POINT('Ctrl Pts',(-0.92278792026947,1.33188468517318,-0.386546956384144));
#10034=CARTESIAN_POINT('Ctrl Pts',(-0.933155485613026,1.35110381617461,
-0.360174810895352));
#10035=CARTESIAN_POINT('Ctrl Pts',(-0.948394987258249,1.39534588636318,
-0.31788699900678));
#10036=CARTESIAN_POINT('Ctrl Pts',(-0.954308486908894,1.42336732874239,
-0.299111603474268));
#10037=CARTESIAN_POINT('Ctrl Pts',(-0.961833761492986,1.48491957299737,
-0.273949373987484));
#10038=CARTESIAN_POINT('Ctrl Pts',(-0.963525491562421,1.5184626473304,-0.267616567329818));
#10039=CARTESIAN_POINT('Ctrl Pts',(-0.963525491562421,1.5815373526696,-0.267616567329818));
#10040=CARTESIAN_POINT('Ctrl Pts',(-0.961833761492986,1.61508042700263,
-0.273949373987484));
#10041=CARTESIAN_POINT('Ctrl Pts',(-0.954308486908894,1.67663267125761,
-0.299111603474268));
#10042=CARTESIAN_POINT('Ctrl Pts',(-0.948394987258249,1.70465411363682,
-0.31788699900678));
#10043=CARTESIAN_POINT('Ctrl Pts',(-0.933155485613026,1.74889618382539,
-0.360174810895352));
#10044=CARTESIAN_POINT('Ctrl Pts',(-0.92278792026947,1.76811531482682,-0.386546956384144));
#10045=CARTESIAN_POINT('Ctrl Pts',(-0.897143218189782,1.79367084275751,
-0.442820664919227));
#10046=CARTESIAN_POINT('Ctrl Pts',(-0.881791875377343,1.8,-0.472691670144998));
#10047=CARTESIAN_POINT('Ctrl Pts',(-0.850258932191534,1.8,-0.527308329855003));
#10048=CARTESIAN_POINT('Ctrl Pts',(-0.832065554235658,1.79367084275751,
-0.555538485325664));
#10049=CARTESIAN_POINT('Ctrl Pts',(-0.796153444118959,1.76811531482682,
-0.605884303066698));
#10050=CARTESIAN_POINT('Ctrl Pts',(-0.778498278845144,1.74889618382539,
-0.62804895077401));
#10051=CARTESIAN_POINT('Ctrl Pts',(-0.749495710301794,1.70465411363682,
-0.662390652284073));
#10052=CARTESIAN_POINT('Ctrl Pts',(-0.73619249062986,1.67663267125761,-0.676899590973058));
#10053=CARTESIAN_POINT('Ctrl Pts',(-0.718163997970498,1.61508042700263,
-0.695997784676728));
#10054=CARTESIAN_POINT('Ctrl Pts',(-0.713525491562421,1.5815373526696,-0.700629269222037));
#10055=CARTESIAN_POINT('Ctrl Pts',(-0.713525491562421,1.55,-0.700629269222037));
#10056=CARTESIAN_POINT('',(-1.28744468918255,1.55,-1.03198167246111));
#10057=CARTESIAN_POINT('',(0.125,1.55,-0.21650635094611));
#10058=CARTESIAN_POINT('',(-1.42894191624432,1.3,-0.825000000000001));
#10059=CARTESIAN_POINT('Ctrl Pts',(-1.42894191624432,1.3,-0.825000000000001));
#10060=CARTESIAN_POINT('Ctrl Pts',(-1.4132207435299,1.3,-0.852229869895949));
#10061=CARTESIAN_POINT('Ctrl Pts',(-1.39561049050871,1.30629366210296,-0.880751161609749));
#10062=CARTESIAN_POINT('Ctrl Pts',(-1.36172049302549,1.33182222741682,-0.932292094146256));
#10063=CARTESIAN_POINT('Ctrl Pts',(-1.34548213209931,1.35105447038507,-0.955340251466735));
#10064=CARTESIAN_POINT('Ctrl Pts',(-1.31917543061769,1.39539254159618,-0.991349264982991));
#10065=CARTESIAN_POINT('Ctrl Pts',(-1.30734972067592,1.42347183818157,-1.00672880483252));
#10066=CARTESIAN_POINT('Ctrl Pts',(-1.29146042158868,1.48505200040818,-1.02703269653942));
#10067=CARTESIAN_POINT('Ctrl Pts',(-1.28744468918255,1.51855708359447,-1.03198167246111));
#10068=CARTESIAN_POINT('Ctrl Pts',(-1.28744468918255,1.55,-1.03198167246111));
#10069=CARTESIAN_POINT('',(-1.42894191624432,1.8,-0.825000000000001));
#10070=CARTESIAN_POINT('Ctrl Pts',(-1.42894191624432,1.8,-0.825000000000001));
#10071=CARTESIAN_POINT('Ctrl Pts',(-1.44466308895875,1.8,-0.797770130104052));
#10072=CARTESIAN_POINT('Ctrl Pts',(-1.46055812562105,1.79370633789704,-0.768258557763732));
#10073=CARTESIAN_POINT('Ctrl Pts',(-1.48824888379079,1.76817777258318,-0.713138492740816));
#10074=CARTESIAN_POINT('Ctrl Pts',(-1.50008999307766,1.74894552961493,-0.687551581002689));
#10075=CARTESIAN_POINT('Ctrl Pts',(-1.51812136280714,1.70460745840382,-0.646764802471699));
#10076=CARTESIAN_POINT('Ctrl Pts',(-1.52552758004446,1.67652816181843,-0.628833667319578));
#10077=CARTESIAN_POINT('Ctrl Pts',(-1.53516661651472,1.61494799959182,-0.60492118480825));
#10078=CARTESIAN_POINT('Ctrl Pts',(-1.53744468918255,1.58144291640553,-0.598968970568896));
#10079=CARTESIAN_POINT('Ctrl Pts',(-1.53744468918255,1.51855708359447,-0.598968970568896));
#10080=CARTESIAN_POINT('Ctrl Pts',(-1.53516661651472,1.48505200040818,-0.60492118480825));
#10081=CARTESIAN_POINT('Ctrl Pts',(-1.52552758004446,1.42347183818157,-0.628833667319578));
#10082=CARTESIAN_POINT('Ctrl Pts',(-1.51812136280714,1.39539254159618,-0.646764802471699));
#10083=CARTESIAN_POINT('Ctrl Pts',(-1.50008999307766,1.35105447038507,-0.687551581002689));
#10084=CARTESIAN_POINT('Ctrl Pts',(-1.48824888379079,1.33182222741682,-0.713138492740816));
#10085=CARTESIAN_POINT('Ctrl Pts',(-1.46055812562105,1.30629366210296,-0.768258557763732));
#10086=CARTESIAN_POINT('Ctrl Pts',(-1.44466308895875,1.3,-0.797770130104052));
#10087=CARTESIAN_POINT('Ctrl Pts',(-1.42894191624432,1.3,-0.825000000000001));
#10088=CARTESIAN_POINT('Ctrl Pts',(-1.28744468918255,1.55,-1.03198167246111));
#10089=CARTESIAN_POINT('Ctrl Pts',(-1.28744468918255,1.58144291640553,-1.03198167246111));
#10090=CARTESIAN_POINT('Ctrl Pts',(-1.29146042158868,1.61494799959182,-1.02703269653942));
#10091=CARTESIAN_POINT('Ctrl Pts',(-1.30734972067592,1.67652816181843,-1.00672880483252));
#10092=CARTESIAN_POINT('Ctrl Pts',(-1.31917543061769,1.70460745840382,-0.991349264982991));
#10093=CARTESIAN_POINT('Ctrl Pts',(-1.34548213209931,1.74894552961493,-0.955340251466734));
#10094=CARTESIAN_POINT('Ctrl Pts',(-1.36172049302549,1.76817777258318,-0.932292094146256));
#10095=CARTESIAN_POINT('Ctrl Pts',(-1.39561049050871,1.79370633789704,-0.880751161609749));
#10096=CARTESIAN_POINT('Ctrl Pts',(-1.4132207435299,1.8,-0.852229869895949));
#10097=CARTESIAN_POINT('Ctrl Pts',(-1.42894191624432,1.8,-0.825000000000001));
#10098=CARTESIAN_POINT('Origin',(0.,1.55,0.));
#10099=CARTESIAN_POINT('',(-1.65,0.85,-2.02066721859313E-16));
#10100=CARTESIAN_POINT('Origin',(0.,0.85,0.));
#10101=CARTESIAN_POINT('',(-1.65,2.25,-2.02066721859313E-16));
#10102=CARTESIAN_POINT('',(-1.65,1.55,-2.02066721859313E-16));
#10103=CARTESIAN_POINT('Origin',(0.,2.25,0.));
#10104=CARTESIAN_POINT('',(-1.42894191624432,1.3,0.825));
#10105=CARTESIAN_POINT('',(-1.42894191624432,1.8,0.825));
#10106=CARTESIAN_POINT('Ctrl Pts',(-1.42894191624432,1.3,0.825));
#10107=CARTESIAN_POINT('Ctrl Pts',(-1.44466308895875,1.3,0.797770130104051));
#10108=CARTESIAN_POINT('Ctrl Pts',(-1.46055812562105,1.30629366210296,0.768258557763731));
#10109=CARTESIAN_POINT('Ctrl Pts',(-1.48824888379079,1.33182222741682,0.713138492740815));
#10110=CARTESIAN_POINT('Ctrl Pts',(-1.50008999307766,1.35105447038507,0.687551581002688));
#10111=CARTESIAN_POINT('Ctrl Pts',(-1.51812136280714,1.39539254159618,0.646764802471698));
#10112=CARTESIAN_POINT('Ctrl Pts',(-1.52552758004446,1.42347183818157,0.628833667319577));
#10113=CARTESIAN_POINT('Ctrl Pts',(-1.53516661651472,1.48505200040818,0.604921184808249));
#10114=CARTESIAN_POINT('Ctrl Pts',(-1.53744468918255,1.51855708359447,0.598968970568895));
#10115=CARTESIAN_POINT('Ctrl Pts',(-1.53744468918255,1.58144291640553,0.598968970568895));
#10116=CARTESIAN_POINT('Ctrl Pts',(-1.53516661651472,1.61494799959182,0.604921184808249));
#10117=CARTESIAN_POINT('Ctrl Pts',(-1.52552758004446,1.67652816181843,0.628833667319577));
#10118=CARTESIAN_POINT('Ctrl Pts',(-1.51812136280714,1.70460745840382,0.646764802471698));
#10119=CARTESIAN_POINT('Ctrl Pts',(-1.50008999307766,1.74894552961493,0.687551581002688));
#10120=CARTESIAN_POINT('Ctrl Pts',(-1.48824888379079,1.76817777258318,0.713138492740815));
#10121=CARTESIAN_POINT('Ctrl Pts',(-1.46055812562105,1.79370633789704,0.768258557763731));
#10122=CARTESIAN_POINT('Ctrl Pts',(-1.44466308895875,1.8,0.797770130104051));
#10123=CARTESIAN_POINT('Ctrl Pts',(-1.42894191624432,1.8,0.825));
#10124=CARTESIAN_POINT('',(-1.28744468918255,1.55,1.03198167246111));
#10125=CARTESIAN_POINT('Ctrl Pts',(-1.42894191624432,1.8,0.825));
#10126=CARTESIAN_POINT('Ctrl Pts',(-1.4132207435299,1.8,0.852229869895948));
#10127=CARTESIAN_POINT('Ctrl Pts',(-1.39561049050871,1.79370633789704,0.880751161609747));
#10128=CARTESIAN_POINT('Ctrl Pts',(-1.36172049302549,1.76817777258318,0.932292094146255));
#10129=CARTESIAN_POINT('Ctrl Pts',(-1.34548213209931,1.74894552961493,0.955340251466733));
#10130=CARTESIAN_POINT('Ctrl Pts',(-1.31917543061769,1.70460745840382,0.991349264982989));
#10131=CARTESIAN_POINT('Ctrl Pts',(-1.30734972067592,1.67652816181843,1.00672880483252));
#10132=CARTESIAN_POINT('Ctrl Pts',(-1.29146042158868,1.61494799959182,1.02703269653942));
#10133=CARTESIAN_POINT('Ctrl Pts',(-1.28744468918255,1.58144291640553,1.03198167246111));
#10134=CARTESIAN_POINT('Ctrl Pts',(-1.28744468918255,1.55,1.03198167246111));
#10135=CARTESIAN_POINT('Ctrl Pts',(-1.28744468918255,1.55,1.03198167246111));
#10136=CARTESIAN_POINT('Ctrl Pts',(-1.28744468918255,1.51855708359447,1.03198167246111));
#10137=CARTESIAN_POINT('Ctrl Pts',(-1.29146042158868,1.48505200040818,1.02703269653942));
#10138=CARTESIAN_POINT('Ctrl Pts',(-1.30734972067592,1.42347183818157,1.00672880483252));
#10139=CARTESIAN_POINT('Ctrl Pts',(-1.31917543061769,1.39539254159618,0.99134926498299));
#10140=CARTESIAN_POINT('Ctrl Pts',(-1.34548213209931,1.35105447038508,0.955340251466733));
#10141=CARTESIAN_POINT('Ctrl Pts',(-1.36172049302549,1.33182222741682,0.932292094146255));
#10142=CARTESIAN_POINT('Ctrl Pts',(-1.39561049050871,1.30629366210296,0.880751161609748));
#10143=CARTESIAN_POINT('Ctrl Pts',(-1.4132207435299,1.3,0.852229869895949));
#10144=CARTESIAN_POINT('Ctrl Pts',(-1.42894191624432,1.3,0.825));
#10145=CARTESIAN_POINT('',(1.42894191624432,1.8,-0.825));
#10146=CARTESIAN_POINT('',(1.42894191624432,1.3,-0.825));
#10147=CARTESIAN_POINT('Ctrl Pts',(1.42894191624432,1.8,-0.825));
#10148=CARTESIAN_POINT('Ctrl Pts',(1.4132207435299,1.8,-0.852229869895949));
#10149=CARTESIAN_POINT('Ctrl Pts',(1.39561049050871,1.79370633789704,-0.880751161609748));
#10150=CARTESIAN_POINT('Ctrl Pts',(1.36172049302549,1.76817777258318,-0.932292094146255));
#10151=CARTESIAN_POINT('Ctrl Pts',(1.34548213209931,1.74894552961493,-0.955340251466734));
#10152=CARTESIAN_POINT('Ctrl Pts',(1.31917543061769,1.70460745840382,-0.99134926498299));
#10153=CARTESIAN_POINT('Ctrl Pts',(1.30734972067592,1.67652816181843,-1.00672880483252));
#10154=CARTESIAN_POINT('Ctrl Pts',(1.29146042158868,1.61494799959182,-1.02703269653942));
#10155=CARTESIAN_POINT('Ctrl Pts',(1.28744468918255,1.58144291640553,-1.03198167246111));
#10156=CARTESIAN_POINT('Ctrl Pts',(1.28744468918255,1.51855708359447,-1.03198167246111));
#10157=CARTESIAN_POINT('Ctrl Pts',(1.29146042158868,1.48505200040818,-1.02703269653942));
#10158=CARTESIAN_POINT('Ctrl Pts',(1.30734972067592,1.42347183818157,-1.00672880483252));
#10159=CARTESIAN_POINT('Ctrl Pts',(1.31917543061769,1.39539254159618,-0.99134926498299));
#10160=CARTESIAN_POINT('Ctrl Pts',(1.34548213209931,1.35105447038507,-0.955340251466734));
#10161=CARTESIAN_POINT('Ctrl Pts',(1.36172049302549,1.33182222741682,-0.932292094146255));
#10162=CARTESIAN_POINT('Ctrl Pts',(1.39561049050871,1.30629366210296,-0.880751161609748));
#10163=CARTESIAN_POINT('Ctrl Pts',(1.4132207435299,1.3,-0.852229869895948));
#10164=CARTESIAN_POINT('Ctrl Pts',(1.42894191624432,1.3,-0.825));
#10165=CARTESIAN_POINT('',(1.53744468918255,1.55,-0.598968970568895));
#10166=CARTESIAN_POINT('Ctrl Pts',(1.42894191624432,1.3,-0.825));
#10167=CARTESIAN_POINT('Ctrl Pts',(1.44466308895875,1.3,-0.797770130104051));
#10168=CARTESIAN_POINT('Ctrl Pts',(1.46055812562105,1.30629366210296,-0.768258557763731));
#10169=CARTESIAN_POINT('Ctrl Pts',(1.48824888379079,1.33182222741682,-0.713138492740815));
#10170=CARTESIAN_POINT('Ctrl Pts',(1.50008999307766,1.35105447038507,-0.687551581002688));
#10171=CARTESIAN_POINT('Ctrl Pts',(1.51812136280714,1.39539254159618,-0.646764802471698));
#10172=CARTESIAN_POINT('Ctrl Pts',(1.52552758004446,1.42347183818157,-0.628833667319577));
#10173=CARTESIAN_POINT('Ctrl Pts',(1.53516661651472,1.48505200040818,-0.604921184808249));
#10174=CARTESIAN_POINT('Ctrl Pts',(1.53744468918255,1.51855708359447,-0.598968970568895));
#10175=CARTESIAN_POINT('Ctrl Pts',(1.53744468918255,1.55,-0.598968970568895));
#10176=CARTESIAN_POINT('Ctrl Pts',(1.53744468918255,1.55,-0.598968970568895));
#10177=CARTESIAN_POINT('Ctrl Pts',(1.53744468918255,1.58144291640553,-0.598968970568895));
#10178=CARTESIAN_POINT('Ctrl Pts',(1.53516661651472,1.61494799959182,-0.604921184808249));
#10179=CARTESIAN_POINT('Ctrl Pts',(1.52552758004446,1.67652816181843,-0.628833667319577));
#10180=CARTESIAN_POINT('Ctrl Pts',(1.51812136280714,1.70460745840382,-0.646764802471698));
#10181=CARTESIAN_POINT('Ctrl Pts',(1.50008999307766,1.74894552961493,-0.687551581002688));
#10182=CARTESIAN_POINT('Ctrl Pts',(1.48824888379079,1.76817777258318,-0.713138492740815));
#10183=CARTESIAN_POINT('Ctrl Pts',(1.46055812562105,1.79370633789704,-0.768258557763731));
#10184=CARTESIAN_POINT('Ctrl Pts',(1.44466308895875,1.8,-0.797770130104051));
#10185=CARTESIAN_POINT('Ctrl Pts',(1.42894191624432,1.8,-0.825));
#10186=CARTESIAN_POINT('',(0.,1.3,-1.65));
#10187=CARTESIAN_POINT('',(0.,1.8,-1.65));
#10188=CARTESIAN_POINT('Ctrl Pts',(1.38777878078145E-17,1.3,-1.65));
#10189=CARTESIAN_POINT('Ctrl Pts',(0.0314423454288489,1.3,-1.65));
#10190=CARTESIAN_POINT('Ctrl Pts',(0.0649476351123396,1.30629366210296,
-1.64900971937348));
#10191=CARTESIAN_POINT('Ctrl Pts',(0.126528390765307,1.33182222741682,-1.64543058688707));
#10192=CARTESIAN_POINT('Ctrl Pts',(0.154607860978348,1.35105447038507,-1.64289183246942));
#10193=CARTESIAN_POINT('Ctrl Pts',(0.198945932189457,1.39539254159618,-1.63811406745469));
#10194=CARTESIAN_POINT('Ctrl Pts',(0.218177859368546,1.42347183818157,-1.63556247215209));
#10195=CARTESIAN_POINT('Ctrl Pts',(0.243706194926033,1.48505200040818,-1.63195388134767));
#10196=CARTESIAN_POINT('Ctrl Pts',(0.25,1.51855708359447,-1.63095064303001));
#10197=CARTESIAN_POINT('Ctrl Pts',(0.25,1.58144291640553,-1.63095064303001));
#10198=CARTESIAN_POINT('Ctrl Pts',(0.243706194926033,1.61494799959182,-1.63195388134767));
#10199=CARTESIAN_POINT('Ctrl Pts',(0.218177859368546,1.67652816181843,-1.63556247215209));
#10200=CARTESIAN_POINT('Ctrl Pts',(0.198945932189457,1.70460745840382,-1.63811406745469));
#10201=CARTESIAN_POINT('Ctrl Pts',(0.154607860978349,1.74894552961493,-1.64289183246942));
#10202=CARTESIAN_POINT('Ctrl Pts',(0.126528390765307,1.76817777258318,-1.64543058688707));
#10203=CARTESIAN_POINT('Ctrl Pts',(0.0649476351123398,1.79370633789704,
-1.64900971937348));
#10204=CARTESIAN_POINT('Ctrl Pts',(0.031442345428849,1.8,-1.65));
#10205=CARTESIAN_POINT('Ctrl Pts',(7.63278329429795E-17,1.8,-1.65));
#10206=CARTESIAN_POINT('',(-0.25,1.55,-1.63095064303001));
#10207=CARTESIAN_POINT('Ctrl Pts',(9.0205620750794E-17,1.8,-1.65));
#10208=CARTESIAN_POINT('Ctrl Pts',(-0.0314423454288488,1.8,-1.65));
#10209=CARTESIAN_POINT('Ctrl Pts',(-0.0649476351123396,1.79370633789704,
-1.64900971937348));
#10210=CARTESIAN_POINT('Ctrl Pts',(-0.126528390765307,1.76817777258318,
-1.64543058688707));
#10211=CARTESIAN_POINT('Ctrl Pts',(-0.154607860978348,1.74894552961493,
-1.64289183246942));
#10212=CARTESIAN_POINT('Ctrl Pts',(-0.198945932189456,1.70460745840382,
-1.63811406745469));
#10213=CARTESIAN_POINT('Ctrl Pts',(-0.218177859368546,1.67652816181843,
-1.63556247215209));
#10214=CARTESIAN_POINT('Ctrl Pts',(-0.243706194926033,1.61494799959182,
-1.63195388134767));
#10215=CARTESIAN_POINT('Ctrl Pts',(-0.25,1.58144291640553,-1.63095064303001));
#10216=CARTESIAN_POINT('Ctrl Pts',(-0.25,1.55,-1.63095064303001));
#10217=CARTESIAN_POINT('Ctrl Pts',(-0.25,1.55,-1.63095064303001));
#10218=CARTESIAN_POINT('Ctrl Pts',(-0.25,1.51855708359447,-1.63095064303001));
#10219=CARTESIAN_POINT('Ctrl Pts',(-0.243706194926033,1.48505200040818,
-1.63195388134767));
#10220=CARTESIAN_POINT('Ctrl Pts',(-0.218177859368546,1.42347183818157,
-1.63556247215209));
#10221=CARTESIAN_POINT('Ctrl Pts',(-0.198945932189457,1.39539254159618,
-1.63811406745469));
#10222=CARTESIAN_POINT('Ctrl Pts',(-0.154607860978349,1.35105447038507,
-1.64289183246942));
#10223=CARTESIAN_POINT('Ctrl Pts',(-0.126528390765307,1.33182222741682,
-1.64543058688707));
#10224=CARTESIAN_POINT('Ctrl Pts',(-0.0649476351123398,1.30629366210296,
-1.64900971937348));
#10225=CARTESIAN_POINT('Ctrl Pts',(-0.031442345428849,1.3,-1.65));
#10226=CARTESIAN_POINT('Ctrl Pts',(-4.85722573273506E-17,1.3,-1.65));
#10227=CARTESIAN_POINT('',(0.,1.8,1.65));
#10228=CARTESIAN_POINT('',(0.,1.3,1.65));
#10229=CARTESIAN_POINT('Ctrl Pts',(8.32667268468867E-17,1.8,1.65));
#10230=CARTESIAN_POINT('Ctrl Pts',(0.031442345428849,1.8,1.65));
#10231=CARTESIAN_POINT('Ctrl Pts',(0.0649476351123398,1.79370633789704,
1.64900971937348));
#10232=CARTESIAN_POINT('Ctrl Pts',(0.126528390765307,1.76817777258318,1.64543058688707));
#10233=CARTESIAN_POINT('Ctrl Pts',(0.154607860978349,1.74894552961493,1.64289183246942));
#10234=CARTESIAN_POINT('Ctrl Pts',(0.198945932189457,1.70460745840382,1.63811406745469));
#10235=CARTESIAN_POINT('Ctrl Pts',(0.218177859368546,1.67652816181843,1.63556247215209));
#10236=CARTESIAN_POINT('Ctrl Pts',(0.243706194926033,1.61494799959182,1.63195388134767));
#10237=CARTESIAN_POINT('Ctrl Pts',(0.25,1.58144291640553,1.63095064303001));
#10238=CARTESIAN_POINT('Ctrl Pts',(0.25,1.51855708359447,1.63095064303001));
#10239=CARTESIAN_POINT('Ctrl Pts',(0.243706194926033,1.48505200040818,1.63195388134767));
#10240=CARTESIAN_POINT('Ctrl Pts',(0.218177859368546,1.42347183818157,1.63556247215209));
#10241=CARTESIAN_POINT('Ctrl Pts',(0.198945932189457,1.39539254159618,1.63811406745469));
#10242=CARTESIAN_POINT('Ctrl Pts',(0.154607860978348,1.35105447038507,1.64289183246942));
#10243=CARTESIAN_POINT('Ctrl Pts',(0.126528390765307,1.33182222741682,1.64543058688707));
#10244=CARTESIAN_POINT('Ctrl Pts',(0.0649476351123397,1.30629366210296,
1.64900971937348));
#10245=CARTESIAN_POINT('Ctrl Pts',(0.0314423454288488,1.3,1.65));
#10246=CARTESIAN_POINT('Ctrl Pts',(-1.38777878078145E-17,1.3,1.65));
#10247=CARTESIAN_POINT('',(-0.25,1.55,1.63095064303001));
#10248=CARTESIAN_POINT('Ctrl Pts',(-5.55111512312578E-17,1.3,1.65));
#10249=CARTESIAN_POINT('Ctrl Pts',(-0.031442345428849,1.3,1.65));
#10250=CARTESIAN_POINT('Ctrl Pts',(-0.0649476351123398,1.30629366210296,
1.64900971937348));
#10251=CARTESIAN_POINT('Ctrl Pts',(-0.126528390765307,1.33182222741682,
1.64543058688707));
#10252=CARTESIAN_POINT('Ctrl Pts',(-0.154607860978349,1.35105447038507,
1.64289183246942));
#10253=CARTESIAN_POINT('Ctrl Pts',(-0.198945932189457,1.39539254159618,
1.63811406745469));
#10254=CARTESIAN_POINT('Ctrl Pts',(-0.218177859368546,1.42347183818157,
1.63556247215209));
#10255=CARTESIAN_POINT('Ctrl Pts',(-0.243706194926033,1.48505200040818,
1.63195388134767));
#10256=CARTESIAN_POINT('Ctrl Pts',(-0.25,1.51855708359447,1.63095064303001));
#10257=CARTESIAN_POINT('Ctrl Pts',(-0.25,1.55,1.63095064303001));
#10258=CARTESIAN_POINT('Ctrl Pts',(-0.25,1.55,1.63095064303001));
#10259=CARTESIAN_POINT('Ctrl Pts',(-0.25,1.58144291640553,1.63095064303001));
#10260=CARTESIAN_POINT('Ctrl Pts',(-0.243706194926033,1.61494799959182,
1.63195388134767));
#10261=CARTESIAN_POINT('Ctrl Pts',(-0.218177859368546,1.67652816181843,
1.63556247215209));
#10262=CARTESIAN_POINT('Ctrl Pts',(-0.198945932189456,1.70460745840382,
1.63811406745469));
#10263=CARTESIAN_POINT('Ctrl Pts',(-0.154607860978348,1.74894552961493,
1.64289183246942));
#10264=CARTESIAN_POINT('Ctrl Pts',(-0.126528390765307,1.76817777258318,
1.64543058688707));
#10265=CARTESIAN_POINT('Ctrl Pts',(-0.0649476351123396,1.79370633789704,
1.64900971937348));
#10266=CARTESIAN_POINT('Ctrl Pts',(-0.0314423454288488,1.8,1.65));
#10267=CARTESIAN_POINT('Ctrl Pts',(7.63278329429795E-17,1.8,1.65));
#10268=CARTESIAN_POINT('Origin',(0.,1.55,0.));
#10269=CARTESIAN_POINT('',(-0.713525491562421,1.55,0.700629269222037));
#10270=CARTESIAN_POINT('',(0.125,1.55,0.21650635094611));
#10271=CARTESIAN_POINT('Ctrl Pts',(-0.713525491562421,1.55,0.700629269222037));
#10272=CARTESIAN_POINT('Ctrl Pts',(-0.713525491562421,1.5815373526696,0.700629269222037));
#10273=CARTESIAN_POINT('Ctrl Pts',(-0.718163997970498,1.61508042700263,
0.695997784676727));
#10274=CARTESIAN_POINT('Ctrl Pts',(-0.73619249062986,1.67663267125761,0.676899590973058));
#10275=CARTESIAN_POINT('Ctrl Pts',(-0.749495710301795,1.70465411363682,
0.662390652284073));
#10276=CARTESIAN_POINT('Ctrl Pts',(-0.778498278845144,1.74889618382539,
0.628048950774009));
#10277=CARTESIAN_POINT('Ctrl Pts',(-0.796153444118959,1.76811531482682,
0.605884303066698));
#10278=CARTESIAN_POINT('Ctrl Pts',(-0.832065554235658,1.79367084275751,
0.555538485325663));
#10279=CARTESIAN_POINT('Ctrl Pts',(-0.850258932191534,1.8,0.527308329855002));
#10280=CARTESIAN_POINT('Ctrl Pts',(-0.881791875377343,1.8,0.472691670144998));
#10281=CARTESIAN_POINT('Ctrl Pts',(-0.897143218189782,1.79367084275751,
0.442820664919227));
#10282=CARTESIAN_POINT('Ctrl Pts',(-0.92278792026947,1.76811531482682,0.386546956384144));
#10283=CARTESIAN_POINT('Ctrl Pts',(-0.933155485613026,1.74889618382539,
0.360174810895352));
#10284=CARTESIAN_POINT('Ctrl Pts',(-0.948394987258249,1.70465411363682,
0.31788699900678));
#10285=CARTESIAN_POINT('Ctrl Pts',(-0.954308486908894,1.67663267125761,
0.299111603474267));
#10286=CARTESIAN_POINT('Ctrl Pts',(-0.961833761492987,1.61508042700263,
0.273949373987484));
#10287=CARTESIAN_POINT('Ctrl Pts',(-0.963525491562421,1.5815373526696,0.267616567329817));
#10288=CARTESIAN_POINT('Ctrl Pts',(-0.963525491562421,1.5184626473304,0.267616567329817));
#10289=CARTESIAN_POINT('Ctrl Pts',(-0.961833761492987,1.48491957299737,
0.273949373987484));
#10290=CARTESIAN_POINT('Ctrl Pts',(-0.954308486908894,1.42336732874239,
0.299111603474267));
#10291=CARTESIAN_POINT('Ctrl Pts',(-0.948394987258249,1.39534588636318,
0.31788699900678));
#10292=CARTESIAN_POINT('Ctrl Pts',(-0.933155485613026,1.35110381617461,
0.360174810895352));
#10293=CARTESIAN_POINT('Ctrl Pts',(-0.92278792026947,1.33188468517318,0.386546956384144));
#10294=CARTESIAN_POINT('Ctrl Pts',(-0.897143218189782,1.30632915724249,
0.442820664919227));
#10295=CARTESIAN_POINT('Ctrl Pts',(-0.881791875377343,1.3,0.472691670144998));
#10296=CARTESIAN_POINT('Ctrl Pts',(-0.850258932191534,1.3,0.527308329855002));
#10297=CARTESIAN_POINT('Ctrl Pts',(-0.832065554235658,1.30632915724249,
0.555538485325663));
#10298=CARTESIAN_POINT('Ctrl Pts',(-0.796153444118959,1.33188468517318,
0.605884303066698));
#10299=CARTESIAN_POINT('Ctrl Pts',(-0.778498278845144,1.35110381617461,
0.628048950774009));
#10300=CARTESIAN_POINT('Ctrl Pts',(-0.749495710301795,1.39534588636318,
0.662390652284073));
#10301=CARTESIAN_POINT('Ctrl Pts',(-0.73619249062986,1.42336732874239,0.676899590973058));
#10302=CARTESIAN_POINT('Ctrl Pts',(-0.718163997970498,1.48491957299737,
0.695997784676727));
#10303=CARTESIAN_POINT('Ctrl Pts',(-0.713525491562421,1.5184626473304,0.700629269222037));
#10304=CARTESIAN_POINT('Ctrl Pts',(-0.713525491562421,1.55,0.700629269222037));
#10305=CARTESIAN_POINT('Origin',(0.,1.55,0.));
#10306=CARTESIAN_POINT('',(0.963525491562421,1.55,-0.267616567329817));
#10307=CARTESIAN_POINT('Ctrl Pts',(0.963525491562421,1.55,-0.267616567329817));
#10308=CARTESIAN_POINT('Ctrl Pts',(0.963525491562421,1.5184626473304,-0.267616567329817));
#10309=CARTESIAN_POINT('Ctrl Pts',(0.961833761492987,1.48491957299737,-0.273949373987484));
#10310=CARTESIAN_POINT('Ctrl Pts',(0.954308486908894,1.42336732874239,-0.299111603474267));
#10311=CARTESIAN_POINT('Ctrl Pts',(0.948394987258249,1.39534588636318,-0.31788699900678));
#10312=CARTESIAN_POINT('Ctrl Pts',(0.933155485613026,1.35110381617461,-0.360174810895352));
#10313=CARTESIAN_POINT('Ctrl Pts',(0.92278792026947,1.33188468517318,-0.386546956384144));
#10314=CARTESIAN_POINT('Ctrl Pts',(0.897143218189782,1.30632915724249,-0.442820664919227));
#10315=CARTESIAN_POINT('Ctrl Pts',(0.881791875377343,1.3,-0.472691670144998));
#10316=CARTESIAN_POINT('Ctrl Pts',(0.850258932191534,1.3,-0.527308329855002));
#10317=CARTESIAN_POINT('Ctrl Pts',(0.832065554235658,1.30632915724249,-0.555538485325663));
#10318=CARTESIAN_POINT('Ctrl Pts',(0.796153444118959,1.33188468517318,-0.605884303066698));
#10319=CARTESIAN_POINT('Ctrl Pts',(0.778498278845144,1.35110381617461,-0.628048950774009));
#10320=CARTESIAN_POINT('Ctrl Pts',(0.749495710301795,1.39534588636318,-0.662390652284073));
#10321=CARTESIAN_POINT('Ctrl Pts',(0.73619249062986,1.42336732874239,-0.676899590973058));
#10322=CARTESIAN_POINT('Ctrl Pts',(0.718163997970498,1.48491957299737,-0.695997784676727));
#10323=CARTESIAN_POINT('Ctrl Pts',(0.713525491562421,1.5184626473304,-0.700629269222037));
#10324=CARTESIAN_POINT('Ctrl Pts',(0.713525491562421,1.5815373526696,-0.700629269222037));
#10325=CARTESIAN_POINT('Ctrl Pts',(0.718163997970498,1.61508042700263,-0.695997784676727));
#10326=CARTESIAN_POINT('Ctrl Pts',(0.73619249062986,1.67663267125761,-0.676899590973058));
#10327=CARTESIAN_POINT('Ctrl Pts',(0.749495710301795,1.70465411363682,-0.662390652284073));
#10328=CARTESIAN_POINT('Ctrl Pts',(0.778498278845144,1.74889618382539,-0.628048950774009));
#10329=CARTESIAN_POINT('Ctrl Pts',(0.796153444118959,1.76811531482682,-0.605884303066698));
#10330=CARTESIAN_POINT('Ctrl Pts',(0.832065554235658,1.79367084275751,-0.555538485325663));
#10331=CARTESIAN_POINT('Ctrl Pts',(0.850258932191534,1.8,-0.527308329855002));
#10332=CARTESIAN_POINT('Ctrl Pts',(0.881791875377343,1.8,-0.472691670144998));
#10333=CARTESIAN_POINT('Ctrl Pts',(0.897143218189782,1.79367084275751,-0.442820664919227));
#10334=CARTESIAN_POINT('Ctrl Pts',(0.92278792026947,1.76811531482682,-0.386546956384144));
#10335=CARTESIAN_POINT('Ctrl Pts',(0.933155485613026,1.74889618382539,-0.360174810895352));
#10336=CARTESIAN_POINT('Ctrl Pts',(0.948394987258249,1.70465411363682,-0.31788699900678));
#10337=CARTESIAN_POINT('Ctrl Pts',(0.954308486908894,1.67663267125761,-0.299111603474267));
#10338=CARTESIAN_POINT('Ctrl Pts',(0.961833761492987,1.61508042700263,-0.273949373987484));
#10339=CARTESIAN_POINT('Ctrl Pts',(0.963525491562421,1.5815373526696,-0.267616567329817));
#10340=CARTESIAN_POINT('Ctrl Pts',(0.963525491562421,1.55,-0.267616567329817));
#10341=CARTESIAN_POINT('',(0.125,1.55,0.21650635094611));
#10342=CARTESIAN_POINT('Origin',(0.,1.55,0.));
#10343=CARTESIAN_POINT('',(-0.25,1.55,-0.968245836551854));
#10344=CARTESIAN_POINT('',(-0.25,1.55,0.));
#10345=CARTESIAN_POINT('Ctrl Pts',(-0.25,1.55,-0.968245836551854));
#10346=CARTESIAN_POINT('Ctrl Pts',(-0.25,1.5815373526696,-0.968245836551854));
#10347=CARTESIAN_POINT('Ctrl Pts',(-0.243669763522489,1.61508042700263,
-0.969947158664211));
#10348=CARTESIAN_POINT('Ctrl Pts',(-0.218115996279034,1.67663267125761,
-0.976011194447325));
#10349=CARTESIAN_POINT('Ctrl Pts',(-0.198899276956455,1.70465411363682,
-0.980277651290853));
#10350=CARTESIAN_POINT('Ctrl Pts',(-0.154657206767882,1.74889618382539,
-0.988223761669361));
#10351=CARTESIAN_POINT('Ctrl Pts',(-0.126634476150511,1.76811531482682,
-0.992431259450842));
#10352=CARTESIAN_POINT('Ctrl Pts',(-0.0650776639541238,1.79367084275751,
-0.99835915024489));
#10353=CARTESIAN_POINT('Ctrl Pts',(-0.0315329431858092,1.8,-1.));
#10354=CARTESIAN_POINT('Ctrl Pts',(0.0315329431858092,1.8,-1.));
#10355=CARTESIAN_POINT('Ctrl Pts',(0.0650776639541238,1.79367084275751,
-0.99835915024489));
#10356=CARTESIAN_POINT('Ctrl Pts',(0.126634476150511,1.76811531482682,-0.992431259450842));
#10357=CARTESIAN_POINT('Ctrl Pts',(0.154657206767882,1.74889618382539,-0.988223761669361));
#10358=CARTESIAN_POINT('Ctrl Pts',(0.198899276956455,1.70465411363682,-0.980277651290853));
#10359=CARTESIAN_POINT('Ctrl Pts',(0.218115996279034,1.67663267125761,-0.976011194447325));
#10360=CARTESIAN_POINT('Ctrl Pts',(0.243669763522488,1.61508042700263,-0.969947158664211));
#10361=CARTESIAN_POINT('Ctrl Pts',(0.25,1.5815373526696,-0.968245836551854));
#10362=CARTESIAN_POINT('Ctrl Pts',(0.25,1.5184626473304,-0.968245836551854));
#10363=CARTESIAN_POINT('Ctrl Pts',(0.243669763522488,1.48491957299737,-0.969947158664211));
#10364=CARTESIAN_POINT('Ctrl Pts',(0.218115996279034,1.42336732874239,-0.976011194447325));
#10365=CARTESIAN_POINT('Ctrl Pts',(0.198899276956455,1.39534588636318,-0.980277651290853));
#10366=CARTESIAN_POINT('Ctrl Pts',(0.154657206767882,1.35110381617461,-0.988223761669361));
#10367=CARTESIAN_POINT('Ctrl Pts',(0.126634476150511,1.33188468517318,-0.992431259450842));
#10368=CARTESIAN_POINT('Ctrl Pts',(0.0650776639541239,1.30632915724249,
-0.99835915024489));
#10369=CARTESIAN_POINT('Ctrl Pts',(0.0315329431858092,1.3,-1.));
#10370=CARTESIAN_POINT('Ctrl Pts',(-0.0315329431858092,1.3,-1.));
#10371=CARTESIAN_POINT('Ctrl Pts',(-0.0650776639541239,1.30632915724249,
-0.99835915024489));
#10372=CARTESIAN_POINT('Ctrl Pts',(-0.126634476150511,1.33188468517318,
-0.992431259450842));
#10373=CARTESIAN_POINT('Ctrl Pts',(-0.154657206767882,1.35110381617461,
-0.988223761669361));
#10374=CARTESIAN_POINT('Ctrl Pts',(-0.198899276956455,1.39534588636318,
-0.980277651290853));
#10375=CARTESIAN_POINT('Ctrl Pts',(-0.218115996279034,1.42336732874239,
-0.976011194447325));
#10376=CARTESIAN_POINT('Ctrl Pts',(-0.243669763522489,1.48491957299737,
-0.969947158664211));
#10377=CARTESIAN_POINT('Ctrl Pts',(-0.25,1.5184626473304,-0.968245836551854));
#10378=CARTESIAN_POINT('Ctrl Pts',(-0.25,1.55,-0.968245836551854));
#10379=CARTESIAN_POINT('Origin',(0.,1.55,0.));
#10380=CARTESIAN_POINT('',(-0.25,1.55,0.968245836551854));
#10381=CARTESIAN_POINT('Ctrl Pts',(-0.25,1.55,0.968245836551854));
#10382=CARTESIAN_POINT('Ctrl Pts',(-0.25,1.5184626473304,0.968245836551854));
#10383=CARTESIAN_POINT('Ctrl Pts',(-0.243669763522489,1.48491957299737,
0.969947158664211));
#10384=CARTESIAN_POINT('Ctrl Pts',(-0.218115996279034,1.42336732874239,
0.976011194447325));
#10385=CARTESIAN_POINT('Ctrl Pts',(-0.198899276956455,1.39534588636318,
0.980277651290853));
#10386=CARTESIAN_POINT('Ctrl Pts',(-0.154657206767882,1.35110381617461,
0.988223761669361));
#10387=CARTESIAN_POINT('Ctrl Pts',(-0.126634476150511,1.33188468517318,
0.992431259450842));
#10388=CARTESIAN_POINT('Ctrl Pts',(-0.065077663954124,1.30632915724249,
0.99835915024489));
#10389=CARTESIAN_POINT('Ctrl Pts',(-0.0315329431858092,1.3,1.));
#10390=CARTESIAN_POINT('Ctrl Pts',(0.0315329431858092,1.3,1.));
#10391=CARTESIAN_POINT('Ctrl Pts',(0.065077663954124,1.30632915724249,0.99835915024489));
#10392=CARTESIAN_POINT('Ctrl Pts',(0.126634476150511,1.33188468517318,0.992431259450842));
#10393=CARTESIAN_POINT('Ctrl Pts',(0.154657206767882,1.35110381617461,0.988223761669361));
#10394=CARTESIAN_POINT('Ctrl Pts',(0.198899276956455,1.39534588636318,0.980277651290853));
#10395=CARTESIAN_POINT('Ctrl Pts',(0.218115996279034,1.42336732874239,0.976011194447325));
#10396=CARTESIAN_POINT('Ctrl Pts',(0.243669763522488,1.48491957299737,0.969947158664211));
#10397=CARTESIAN_POINT('Ctrl Pts',(0.25,1.5184626473304,0.968245836551854));
#10398=CARTESIAN_POINT('Ctrl Pts',(0.25,1.5815373526696,0.968245836551854));
#10399=CARTESIAN_POINT('Ctrl Pts',(0.243669763522488,1.61508042700263,0.969947158664211));
#10400=CARTESIAN_POINT('Ctrl Pts',(0.218115996279034,1.67663267125761,0.976011194447325));
#10401=CARTESIAN_POINT('Ctrl Pts',(0.198899276956455,1.70465411363682,0.980277651290853));
#10402=CARTESIAN_POINT('Ctrl Pts',(0.154657206767882,1.74889618382539,0.988223761669361));
#10403=CARTESIAN_POINT('Ctrl Pts',(0.126634476150511,1.76811531482682,0.992431259450842));
#10404=CARTESIAN_POINT('Ctrl Pts',(0.0650776639541239,1.79367084275751,
0.99835915024489));
#10405=CARTESIAN_POINT('Ctrl Pts',(0.0315329431858092,1.8,1.));
#10406=CARTESIAN_POINT('Ctrl Pts',(-0.0315329431858092,1.8,1.));
#10407=CARTESIAN_POINT('Ctrl Pts',(-0.0650776639541239,1.79367084275751,
0.99835915024489));
#10408=CARTESIAN_POINT('Ctrl Pts',(-0.126634476150511,1.76811531482682,
0.992431259450842));
#10409=CARTESIAN_POINT('Ctrl Pts',(-0.154657206767882,1.74889618382539,
0.988223761669361));
#10410=CARTESIAN_POINT('Ctrl Pts',(-0.198899276956455,1.70465411363682,
0.980277651290853));
#10411=CARTESIAN_POINT('Ctrl Pts',(-0.218115996279034,1.67663267125761,
0.976011194447325));
#10412=CARTESIAN_POINT('Ctrl Pts',(-0.243669763522489,1.61508042700263,
0.969947158664211));
#10413=CARTESIAN_POINT('Ctrl Pts',(-0.25,1.5815373526696,0.968245836551854));
#10414=CARTESIAN_POINT('Ctrl Pts',(-0.25,1.55,0.968245836551854));
#10415=CARTESIAN_POINT('',(-0.25,1.55,0.));
#10416=CARTESIAN_POINT('Origin',(1.65,2.25,0.));
#10417=CARTESIAN_POINT('',(-1.,2.25,-1.22464679914735E-16));
#10418=CARTESIAN_POINT('Origin',(0.,2.25,0.));
#10419=CARTESIAN_POINT('Origin',(1.75,0.85,0.));
#10420=CARTESIAN_POINT('',(-1.75,0.85,-2.14313189850787E-16));
#10421=CARTESIAN_POINT('Origin',(0.,0.85,0.));
#10422=CARTESIAN_POINT('Origin',(0.,0.,0.));
#10423=CARTESIAN_POINT('',(-1.75,-0.85,-2.14313189850787E-16));
#10424=CARTESIAN_POINT('Origin',(0.,-0.85,0.));
#10425=CARTESIAN_POINT('',(-1.75,0.,-2.14313189850787E-16));
#10426=CARTESIAN_POINT('Origin',(1.,-0.85,0.));
#10427=CARTESIAN_POINT('',(-1.,-0.85,-1.22464679914735E-16));
#10428=CARTESIAN_POINT('Origin',(0.,-0.85,0.));
#10429=CARTESIAN_POINT('Origin',(0.,0.7,0.));
#10430=CARTESIAN_POINT('',(-1.,0.7,-1.22464679914735E-16));
#11741=UNCERTAINTY_MEASURE_WITH_UNIT(LENGTH_MEASURE(0.001),#11802,
'DISTANCE_ACCURACY_VALUE',
'Maximum model space distance between geometric entities at asserted c
onnectivities');
#11761=UNCERTAINTY_MEASURE_WITH_UNIT(LENGTH_MEASURE(0.001),#11802,
'DISTANCE_ACCURACY_VALUE',
'Maximum model space distance between geometric entities at asserted c
onnectivities');
#11781=(
GEOMETRIC_REPRESENTATION_CONTEXT(3)
GLOBAL_UNCERTAINTY_ASSIGNED_CONTEXT((#11741))
GLOBAL_UNIT_ASSIGNED_CONTEXT((#11802,#11804,#11805))
REPRESENTATION_CONTEXT('','3D')
);
#11801=(
GEOMETRIC_REPRESENTATION_CONTEXT(3)
GLOBAL_UNCERTAINTY_ASSIGNED_CONTEXT((#11761))
GLOBAL_UNIT_ASSIGNED_CONTEXT((#11802,#11804,#11805))
REPRESENTATION_CONTEXT('','3D')
);
#11802=(
LENGTH_UNIT()
NAMED_UNIT(*)
SI_UNIT(.CENTI.,.METRE.)
);
#11804=(
NAMED_UNIT(*)
PLANE_ANGLE_UNIT()
SI_UNIT($,.RADIAN.)
);
#11805=(
NAMED_UNIT(*)
SI_UNIT($,.STERADIAN.)
SOLID_ANGLE_UNIT()
);
#11825=SHAPE_DEFINITION_REPRESENTATION(#11864,#11964);
#11864=PRODUCT_DEFINITION_SHAPE('',$,#12004);
#11964=SHAPE_REPRESENTATION('',(#6962),#11781);
#11984=PRODUCT_DEFINITION_CONTEXT('part definition',#12103,'design');
#12004=PRODUCT_DEFINITION('Insert bearing','Insert bearing',#12043,#11984);
#12043=PRODUCT_DEFINITION_FORMATION('',$,#12124);
#12103=APPLICATION_CONTEXT(
'Core Data for Automotive Mechanical Design Process');
#12104=PRODUCT_CONTEXT('part definition',#12103,'mechanical');
#12124=PRODUCT('Insert bearing','Insert bearing','Insert bearing',(#12104));
#12207=COLOUR_RGB('Grey',0.48,0.52,0.57);
#12208=FILL_AREA_STYLE_COLOUR('',#12207);
#12209=FILL_AREA_STYLE('',(#12208));
#12210=SURFACE_STYLE_FILL_AREA(#12209);
#12211=SURFACE_SIDE_STYLE('',(#12210));
#12212=SURFACE_STYLE_USAGE(.BOTH.,#12211);
#12213=PRESENTATION_STYLE_ASSIGNMENT((#12212));
ENDSEC;
END-ISO-10303-21;
